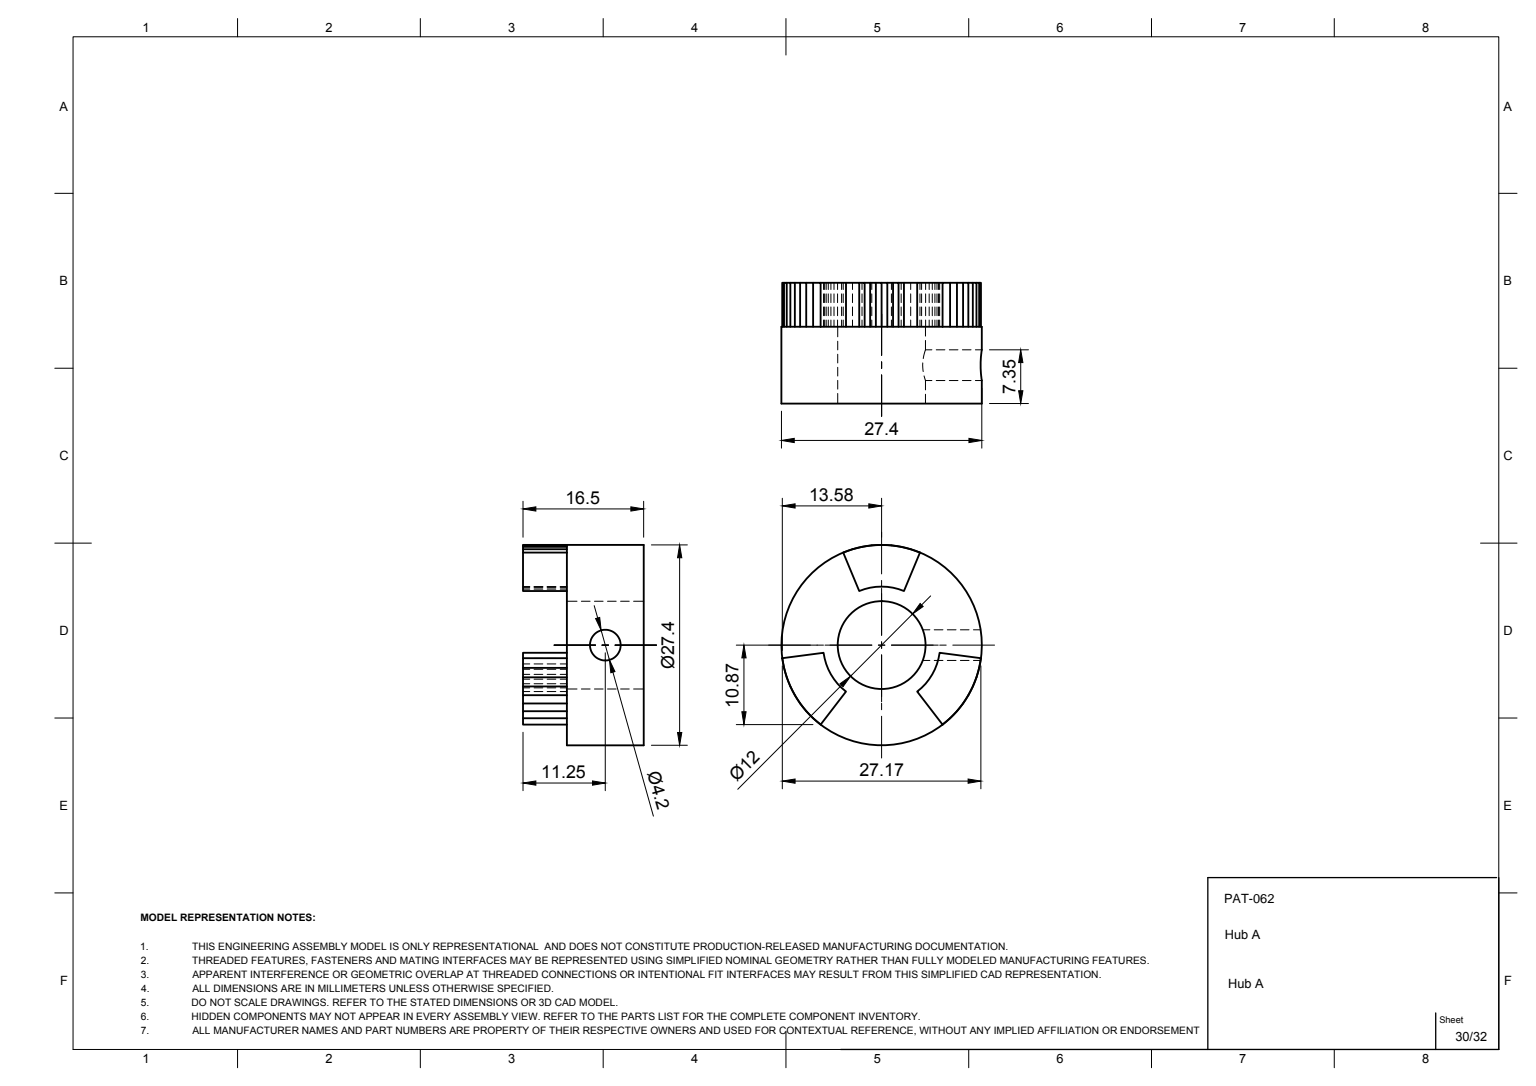
ISO-10303-21;
HEADER;
/* Generated by software containing ST-Developer
 * from STEP Tools, Inc. (www.steptools.com) 
 */

FILE_DESCRIPTION(
/* description */ ('Jaw-coupled motor to shaft test stand'),
/* implementation_level */ '2;1');

FILE_NAME(
/* name */ 'Hub A.step',
/* time_stamp */ '2026-10-27T10:46:06-07:00',
/* author */ (''),
/* organization */ (''),
/* preprocessor_version */ 'ST-DEVELOPER v20.2',
/* originating_system */ 'Autodesk Translation Framework v15.17.0.0',
/* authorisation */ '');

FILE_SCHEMA (('AUTOMOTIVE_DESIGN { 1 0 10303 214 3 1 1 }'));
ENDSEC;

DATA;
#10=MECHANICAL_DESIGN_GEOMETRIC_PRESENTATION_REPRESENTATION('',(#367),#19361);
#267=B_SPLINE_CURVE_WITH_KNOTS('',3,(#17316,#17317,#17318,#17319,#17320,
#17321,#17322,#17323,#17324,#17325,#17326,#17327,#17328,#17329,#17330,#17331,
#17332,#17333),.UNSPECIFIED.,.F.,.F.,(4,2,2,2,2,2,2,2,4),(0.,0.0798638474423531,
0.159727694884706,0.239545993340072,0.319364291795438,0.399182590250804,
0.47900088870617,0.558864736148523,0.638728583590876),.UNSPECIFIED.);
#268=B_SPLINE_CURVE_WITH_KNOTS('',3,(#17334,#17335,#17336,#17337,#17338,
#17339,#17340,#17341,#17342,#17343,#17344,#17345,#17346,#17347,#17348,#17349,
#17350,#17351),.UNSPECIFIED.,.F.,.F.,(4,2,2,2,2,2,2,2,4),(0.638728583590876,
0.718592431033229,0.798456278475582,0.878274576930948,0.958092875386314,
1.03791117384168,1.11772947229705,1.1975933197394,1.27745716718175),
 .UNSPECIFIED.);
#269=B_SPLINE_CURVE_WITH_KNOTS('',3,(#17354,#17355,#17356,#17357,#17358,
#17359,#17360,#17361,#17362,#17363,#17364,#17365,#17366,#17367,#17368,#17369,
#17370,#17371,#17372,#17373,#17374,#17375,#17376,#17377,#17378,#17379,#17380,
#17381,#17382,#17383,#17384,#17385,#17386,#17387),.UNSPECIFIED.,.T.,.F.,
(4,2,2,2,2,2,2,2,2,2,2,2,2,2,2,2,4),(0.,0.079239302416133,0.158478604832266,
0.237716399152057,0.316954193471848,0.39619198779164,0.475429782111431,
0.554669084527564,0.633908386943697,0.71314768935983,0.792386991775963,
0.871624786095754,0.950862580415545,1.03010037473534,1.10933816905513,1.18857747147126,
1.26781677388739),.UNSPECIFIED.);
#302=SHAPE_REPRESENTATION_RELATIONSHIP('SRR','None',#19519,#334);
#334=ADVANCED_BREP_SHAPE_REPRESENTATION('',(#398),#19355);
#367=STYLED_ITEM('',(#19739),#398);
#398=MANIFOLD_SOLID_BREP('Body1',#11013);
#506=FACE_BOUND('',#2012,.T.);
#507=FACE_BOUND('',#2041,.T.);
#508=FACE_BOUND('',#2097,.T.);
#509=FACE_BOUND('',#2099,.T.);
#694=PLANE('',#11869);
#695=PLANE('',#11870);
#696=PLANE('',#11871);
#697=PLANE('',#11872);
#698=PLANE('',#11873);
#699=PLANE('',#11874);
#700=PLANE('',#11875);
#701=PLANE('',#11876);
#702=PLANE('',#11877);
#703=PLANE('',#11878);
#704=PLANE('',#11879);
#705=PLANE('',#11880);
#706=PLANE('',#11881);
#707=PLANE('',#11882);
#708=PLANE('',#11883);
#709=PLANE('',#11884);
#710=PLANE('',#11885);
#711=PLANE('',#11886);
#712=PLANE('',#11887);
#713=PLANE('',#11888);
#714=PLANE('',#11890);
#715=PLANE('',#11892);
#716=PLANE('',#11894);
#717=PLANE('',#11896);
#718=PLANE('',#11898);
#719=PLANE('',#11900);
#720=PLANE('',#11902);
#721=PLANE('',#11904);
#722=PLANE('',#11909);
#723=PLANE('',#11910);
#724=PLANE('',#11911);
#725=PLANE('',#11912);
#726=PLANE('',#11913);
#727=PLANE('',#11914);
#728=PLANE('',#11915);
#729=PLANE('',#11916);
#730=PLANE('',#11917);
#731=PLANE('',#11918);
#732=PLANE('',#11919);
#733=PLANE('',#11920);
#734=PLANE('',#11921);
#735=PLANE('',#11922);
#736=PLANE('',#11923);
#737=PLANE('',#11924);
#738=PLANE('',#11925);
#739=PLANE('',#11926);
#740=PLANE('',#11927);
#741=PLANE('',#11928);
#742=PLANE('',#11930);
#743=PLANE('',#11932);
#744=PLANE('',#11934);
#745=PLANE('',#11936);
#746=PLANE('',#11938);
#747=PLANE('',#11940);
#748=PLANE('',#11942);
#749=PLANE('',#11944);
#750=PLANE('',#11945);
#751=PLANE('',#11946);
#752=PLANE('',#11947);
#753=PLANE('',#11948);
#754=PLANE('',#11949);
#755=PLANE('',#11950);
#756=PLANE('',#11951);
#757=PLANE('',#11952);
#758=PLANE('',#11953);
#759=PLANE('',#11954);
#760=PLANE('',#11955);
#761=PLANE('',#11956);
#762=PLANE('',#11957);
#763=PLANE('',#11958);
#764=PLANE('',#11959);
#765=PLANE('',#11960);
#766=PLANE('',#11961);
#767=PLANE('',#11962);
#768=PLANE('',#11963);
#769=PLANE('',#11965);
#770=PLANE('',#11967);
#771=PLANE('',#11969);
#772=PLANE('',#11971);
#773=PLANE('',#11973);
#774=PLANE('',#11975);
#775=PLANE('',#11977);
#776=PLANE('',#11981);
#1287=FACE_OUTER_BOUND('',#2010,.T.);
#1288=FACE_OUTER_BOUND('',#2011,.T.);
#1289=FACE_OUTER_BOUND('',#2013,.T.);
#1290=FACE_OUTER_BOUND('',#2014,.T.);
#1291=FACE_OUTER_BOUND('',#2015,.T.);
#1292=FACE_OUTER_BOUND('',#2016,.T.);
#1293=FACE_OUTER_BOUND('',#2017,.T.);
#1294=FACE_OUTER_BOUND('',#2018,.T.);
#1295=FACE_OUTER_BOUND('',#2019,.T.);
#1296=FACE_OUTER_BOUND('',#2020,.T.);
#1297=FACE_OUTER_BOUND('',#2021,.T.);
#1298=FACE_OUTER_BOUND('',#2022,.T.);
#1299=FACE_OUTER_BOUND('',#2023,.T.);
#1300=FACE_OUTER_BOUND('',#2024,.T.);
#1301=FACE_OUTER_BOUND('',#2025,.T.);
#1302=FACE_OUTER_BOUND('',#2026,.T.);
#1303=FACE_OUTER_BOUND('',#2027,.T.);
#1304=FACE_OUTER_BOUND('',#2028,.T.);
#1305=FACE_OUTER_BOUND('',#2029,.T.);
#1306=FACE_OUTER_BOUND('',#2030,.T.);
#1307=FACE_OUTER_BOUND('',#2031,.T.);
#1308=FACE_OUTER_BOUND('',#2032,.T.);
#1309=FACE_OUTER_BOUND('',#2033,.T.);
#1310=FACE_OUTER_BOUND('',#2034,.T.);
#1311=FACE_OUTER_BOUND('',#2035,.T.);
#1312=FACE_OUTER_BOUND('',#2036,.T.);
#1313=FACE_OUTER_BOUND('',#2037,.T.);
#1314=FACE_OUTER_BOUND('',#2038,.T.);
#1315=FACE_OUTER_BOUND('',#2039,.T.);
#1316=FACE_OUTER_BOUND('',#2040,.T.);
#1317=FACE_OUTER_BOUND('',#2042,.T.);
#1318=FACE_OUTER_BOUND('',#2043,.T.);
#1319=FACE_OUTER_BOUND('',#2044,.T.);
#1320=FACE_OUTER_BOUND('',#2045,.T.);
#1321=FACE_OUTER_BOUND('',#2046,.T.);
#1322=FACE_OUTER_BOUND('',#2047,.T.);
#1323=FACE_OUTER_BOUND('',#2048,.T.);
#1324=FACE_OUTER_BOUND('',#2049,.T.);
#1325=FACE_OUTER_BOUND('',#2050,.T.);
#1326=FACE_OUTER_BOUND('',#2051,.T.);
#1327=FACE_OUTER_BOUND('',#2052,.T.);
#1328=FACE_OUTER_BOUND('',#2053,.T.);
#1329=FACE_OUTER_BOUND('',#2054,.T.);
#1330=FACE_OUTER_BOUND('',#2055,.T.);
#1331=FACE_OUTER_BOUND('',#2056,.T.);
#1332=FACE_OUTER_BOUND('',#2057,.T.);
#1333=FACE_OUTER_BOUND('',#2058,.T.);
#1334=FACE_OUTER_BOUND('',#2059,.T.);
#1335=FACE_OUTER_BOUND('',#2060,.T.);
#1336=FACE_OUTER_BOUND('',#2061,.T.);
#1337=FACE_OUTER_BOUND('',#2062,.T.);
#1338=FACE_OUTER_BOUND('',#2063,.T.);
#1339=FACE_OUTER_BOUND('',#2064,.T.);
#1340=FACE_OUTER_BOUND('',#2065,.T.);
#1341=FACE_OUTER_BOUND('',#2066,.T.);
#1342=FACE_OUTER_BOUND('',#2067,.T.);
#1343=FACE_OUTER_BOUND('',#2068,.T.);
#1344=FACE_OUTER_BOUND('',#2069,.T.);
#1345=FACE_OUTER_BOUND('',#2070,.T.);
#1346=FACE_OUTER_BOUND('',#2071,.T.);
#1347=FACE_OUTER_BOUND('',#2072,.T.);
#1348=FACE_OUTER_BOUND('',#2073,.T.);
#1349=FACE_OUTER_BOUND('',#2074,.T.);
#1350=FACE_OUTER_BOUND('',#2075,.T.);
#1351=FACE_OUTER_BOUND('',#2076,.T.);
#1352=FACE_OUTER_BOUND('',#2077,.T.);
#1353=FACE_OUTER_BOUND('',#2078,.T.);
#1354=FACE_OUTER_BOUND('',#2079,.T.);
#1355=FACE_OUTER_BOUND('',#2080,.T.);
#1356=FACE_OUTER_BOUND('',#2081,.T.);
#1357=FACE_OUTER_BOUND('',#2082,.T.);
#1358=FACE_OUTER_BOUND('',#2083,.T.);
#1359=FACE_OUTER_BOUND('',#2084,.T.);
#1360=FACE_OUTER_BOUND('',#2085,.T.);
#1361=FACE_OUTER_BOUND('',#2086,.T.);
#1362=FACE_OUTER_BOUND('',#2087,.T.);
#1363=FACE_OUTER_BOUND('',#2088,.T.);
#1364=FACE_OUTER_BOUND('',#2089,.T.);
#1365=FACE_OUTER_BOUND('',#2090,.T.);
#1366=FACE_OUTER_BOUND('',#2091,.T.);
#1367=FACE_OUTER_BOUND('',#2092,.T.);
#1368=FACE_OUTER_BOUND('',#2093,.T.);
#1369=FACE_OUTER_BOUND('',#2094,.T.);
#1370=FACE_OUTER_BOUND('',#2095,.T.);
#1371=FACE_OUTER_BOUND('',#2096,.T.);
#1372=FACE_OUTER_BOUND('',#2098,.T.);
#2010=EDGE_LOOP('',(#8474,#8475,#8476,#8477,#8478));
#2011=EDGE_LOOP('',(#8479,#8480,#8481,#8482));
#2012=EDGE_LOOP('',(#8483,#8484));
#2013=EDGE_LOOP('',(#8485,#8486,#8487,#8488));
#2014=EDGE_LOOP('',(#8489,#8490,#8491,#8492));
#2015=EDGE_LOOP('',(#8493,#8494,#8495,#8496));
#2016=EDGE_LOOP('',(#8497,#8498,#8499,#8500));
#2017=EDGE_LOOP('',(#8501,#8502,#8503,#8504));
#2018=EDGE_LOOP('',(#8505,#8506,#8507,#8508));
#2019=EDGE_LOOP('',(#8509,#8510,#8511,#8512));
#2020=EDGE_LOOP('',(#8513,#8514,#8515,#8516));
#2021=EDGE_LOOP('',(#8517,#8518,#8519,#8520));
#2022=EDGE_LOOP('',(#8521,#8522,#8523,#8524));
#2023=EDGE_LOOP('',(#8525,#8526,#8527,#8528));
#2024=EDGE_LOOP('',(#8529,#8530,#8531,#8532));
#2025=EDGE_LOOP('',(#8533,#8534,#8535,#8536));
#2026=EDGE_LOOP('',(#8537,#8538,#8539,#8540));
#2027=EDGE_LOOP('',(#8541,#8542,#8543,#8544));
#2028=EDGE_LOOP('',(#8545,#8546,#8547,#8548));
#2029=EDGE_LOOP('',(#8549,#8550,#8551,#8552));
#2030=EDGE_LOOP('',(#8553,#8554,#8555,#8556));
#2031=EDGE_LOOP('',(#8557,#8558,#8559,#8560,#8561,#8562,#8563,#8564,#8565,
#8566,#8567,#8568,#8569,#8570,#8571,#8572,#8573,#8574));
#2032=EDGE_LOOP('',(#8575,#8576));
#2033=EDGE_LOOP('',(#8577,#8578));
#2034=EDGE_LOOP('',(#8579,#8580));
#2035=EDGE_LOOP('',(#8581,#8582));
#2036=EDGE_LOOP('',(#8583,#8584));
#2037=EDGE_LOOP('',(#8585,#8586));
#2038=EDGE_LOOP('',(#8587,#8588));
#2039=EDGE_LOOP('',(#8589,#8590));
#2040=EDGE_LOOP('',(#8591,#8592,#8593,#8594,#8595,#8596,#8597,#8598,#8599,
#8600,#8601,#8602,#8603,#8604,#8605,#8606,#8607,#8608,#8609,#8610,#8611,
#8612,#8613,#8614,#8615,#8616,#8617,#8618,#8619,#8620,#8621,#8622,#8623,
#8624));
#2041=EDGE_LOOP('',(#8625));
#2042=EDGE_LOOP('',(#8626,#8627,#8628,#8629));
#2043=EDGE_LOOP('',(#8630,#8631,#8632,#8633));
#2044=EDGE_LOOP('',(#8634,#8635,#8636,#8637));
#2045=EDGE_LOOP('',(#8638,#8639,#8640,#8641));
#2046=EDGE_LOOP('',(#8642,#8643,#8644,#8645));
#2047=EDGE_LOOP('',(#8646,#8647,#8648,#8649));
#2048=EDGE_LOOP('',(#8650,#8651,#8652,#8653));
#2049=EDGE_LOOP('',(#8654,#8655,#8656,#8657));
#2050=EDGE_LOOP('',(#8658,#8659,#8660,#8661));
#2051=EDGE_LOOP('',(#8662,#8663,#8664,#8665));
#2052=EDGE_LOOP('',(#8666,#8667,#8668,#8669));
#2053=EDGE_LOOP('',(#8670,#8671,#8672,#8673));
#2054=EDGE_LOOP('',(#8674,#8675,#8676,#8677));
#2055=EDGE_LOOP('',(#8678,#8679,#8680,#8681));
#2056=EDGE_LOOP('',(#8682,#8683,#8684,#8685));
#2057=EDGE_LOOP('',(#8686,#8687,#8688,#8689));
#2058=EDGE_LOOP('',(#8690,#8691,#8692,#8693));
#2059=EDGE_LOOP('',(#8694,#8695,#8696,#8697));
#2060=EDGE_LOOP('',(#8698,#8699,#8700,#8701,#8702,#8703,#8704,#8705,#8706,
#8707,#8708,#8709,#8710,#8711,#8712,#8713,#8714,#8715));
#2061=EDGE_LOOP('',(#8716,#8717));
#2062=EDGE_LOOP('',(#8718,#8719));
#2063=EDGE_LOOP('',(#8720,#8721));
#2064=EDGE_LOOP('',(#8722,#8723));
#2065=EDGE_LOOP('',(#8724,#8725));
#2066=EDGE_LOOP('',(#8726,#8727));
#2067=EDGE_LOOP('',(#8728,#8729));
#2068=EDGE_LOOP('',(#8730,#8731));
#2069=EDGE_LOOP('',(#8732,#8733,#8734,#8735));
#2070=EDGE_LOOP('',(#8736,#8737,#8738,#8739));
#2071=EDGE_LOOP('',(#8740,#8741,#8742,#8743));
#2072=EDGE_LOOP('',(#8744,#8745,#8746,#8747));
#2073=EDGE_LOOP('',(#8748,#8749,#8750,#8751));
#2074=EDGE_LOOP('',(#8752,#8753,#8754,#8755));
#2075=EDGE_LOOP('',(#8756,#8757,#8758,#8759));
#2076=EDGE_LOOP('',(#8760,#8761,#8762,#8763));
#2077=EDGE_LOOP('',(#8764,#8765,#8766,#8767));
#2078=EDGE_LOOP('',(#8768,#8769,#8770,#8771));
#2079=EDGE_LOOP('',(#8772,#8773,#8774,#8775));
#2080=EDGE_LOOP('',(#8776,#8777,#8778,#8779));
#2081=EDGE_LOOP('',(#8780,#8781,#8782,#8783));
#2082=EDGE_LOOP('',(#8784,#8785,#8786,#8787));
#2083=EDGE_LOOP('',(#8788,#8789,#8790,#8791));
#2084=EDGE_LOOP('',(#8792,#8793,#8794,#8795));
#2085=EDGE_LOOP('',(#8796,#8797,#8798,#8799));
#2086=EDGE_LOOP('',(#8800,#8801,#8802,#8803));
#2087=EDGE_LOOP('',(#8804,#8805,#8806,#8807,#8808,#8809,#8810,#8811,#8812,
#8813,#8814,#8815,#8816,#8817,#8818,#8819,#8820,#8821));
#2088=EDGE_LOOP('',(#8822,#8823));
#2089=EDGE_LOOP('',(#8824,#8825));
#2090=EDGE_LOOP('',(#8826,#8827));
#2091=EDGE_LOOP('',(#8828,#8829));
#2092=EDGE_LOOP('',(#8830,#8831));
#2093=EDGE_LOOP('',(#8832,#8833));
#2094=EDGE_LOOP('',(#8834,#8835));
#2095=EDGE_LOOP('',(#8836,#8837));
#2096=EDGE_LOOP('',(#8838,#8839,#8840,#8841,#8842,#8843,#8844,#8845,#8846,
#8847,#8848,#8849,#8850,#8851,#8852,#8853,#8854,#8855,#8856,#8857,#8858,
#8859,#8860,#8861,#8862,#8863,#8864,#8865,#8866,#8867,#8868));
#2097=EDGE_LOOP('',(#8869));
#2098=EDGE_LOOP('',(#8870));
#2099=EDGE_LOOP('',(#8871));
#2731=LINE('',#17353,#3884);
#2732=LINE('',#17392,#3885);
#2733=LINE('',#17397,#3886);
#2734=LINE('',#17399,#3887);
#2735=LINE('',#17401,#3888);
#2736=LINE('',#17402,#3889);
#2737=LINE('',#17405,#3890);
#2738=LINE('',#17407,#3891);
#2739=LINE('',#17408,#3892);
#2740=LINE('',#17411,#3893);
#2741=LINE('',#17413,#3894);
#2742=LINE('',#17414,#3895);
#2743=LINE('',#17417,#3896);
#2744=LINE('',#17419,#3897);
#2745=LINE('',#17420,#3898);
#2746=LINE('',#17423,#3899);
#2747=LINE('',#17425,#3900);
#2748=LINE('',#17426,#3901);
#2749=LINE('',#17429,#3902);
#2750=LINE('',#17431,#3903);
#2751=LINE('',#17432,#3904);
#2752=LINE('',#17435,#3905);
#2753=LINE('',#17437,#3906);
#2754=LINE('',#17438,#3907);
#2755=LINE('',#17441,#3908);
#2756=LINE('',#17443,#3909);
#2757=LINE('',#17444,#3910);
#2758=LINE('',#17447,#3911);
#2759=LINE('',#17449,#3912);
#2760=LINE('',#17450,#3913);
#2761=LINE('',#17453,#3914);
#2762=LINE('',#17455,#3915);
#2763=LINE('',#17456,#3916);
#2764=LINE('',#17459,#3917);
#2765=LINE('',#17461,#3918);
#2766=LINE('',#17462,#3919);
#2767=LINE('',#17465,#3920);
#2768=LINE('',#17467,#3921);
#2769=LINE('',#17468,#3922);
#2770=LINE('',#17471,#3923);
#2771=LINE('',#17473,#3924);
#2772=LINE('',#17474,#3925);
#2773=LINE('',#17477,#3926);
#2774=LINE('',#17479,#3927);
#2775=LINE('',#17480,#3928);
#2776=LINE('',#17483,#3929);
#2777=LINE('',#17485,#3930);
#2778=LINE('',#17486,#3931);
#2779=LINE('',#17489,#3932);
#2780=LINE('',#17491,#3933);
#2781=LINE('',#17492,#3934);
#2782=LINE('',#17495,#3935);
#2783=LINE('',#17497,#3936);
#2784=LINE('',#17498,#3937);
#2785=LINE('',#17500,#3938);
#2786=LINE('',#17501,#3939);
#2787=LINE('',#17523,#3940);
#2788=LINE('',#17525,#3941);
#2789=LINE('',#17527,#3942);
#2790=LINE('',#17529,#3943);
#2791=LINE('',#17531,#3944);
#2792=LINE('',#17533,#3945);
#2793=LINE('',#17535,#3946);
#2794=LINE('',#17537,#3947);
#2795=LINE('',#17539,#3948);
#2796=LINE('',#17541,#3949);
#2797=LINE('',#17545,#3950);
#2798=LINE('',#17547,#3951);
#2799=LINE('',#17549,#3952);
#2800=LINE('',#17551,#3953);
#2801=LINE('',#17553,#3954);
#2802=LINE('',#17555,#3955);
#2803=LINE('',#17557,#3956);
#2804=LINE('',#17559,#3957);
#2805=LINE('',#17561,#3958);
#2806=LINE('',#17563,#3959);
#2807=LINE('',#17570,#3960);
#2808=LINE('',#17571,#3961);
#2809=LINE('',#17573,#3962);
#2810=LINE('',#17574,#3963);
#2811=LINE('',#17577,#3964);
#2812=LINE('',#17579,#3965);
#2813=LINE('',#17580,#3966);
#2814=LINE('',#17583,#3967);
#2815=LINE('',#17585,#3968);
#2816=LINE('',#17586,#3969);
#2817=LINE('',#17589,#3970);
#2818=LINE('',#17591,#3971);
#2819=LINE('',#17592,#3972);
#2820=LINE('',#17595,#3973);
#2821=LINE('',#17597,#3974);
#2822=LINE('',#17598,#3975);
#2823=LINE('',#17601,#3976);
#2824=LINE('',#17603,#3977);
#2825=LINE('',#17604,#3978);
#2826=LINE('',#17607,#3979);
#2827=LINE('',#17609,#3980);
#2828=LINE('',#17610,#3981);
#2829=LINE('',#17613,#3982);
#2830=LINE('',#17614,#3983);
#2831=LINE('',#17615,#3984);
#2832=LINE('',#17618,#3985);
#2833=LINE('',#17619,#3986);
#2834=LINE('',#17622,#3987);
#2835=LINE('',#17623,#3988);
#2836=LINE('',#17626,#3989);
#2837=LINE('',#17627,#3990);
#2838=LINE('',#17630,#3991);
#2839=LINE('',#17631,#3992);
#2840=LINE('',#17634,#3993);
#2841=LINE('',#17635,#3994);
#2842=LINE('',#17638,#3995);
#2843=LINE('',#17639,#3996);
#2844=LINE('',#17642,#3997);
#2845=LINE('',#17643,#3998);
#2846=LINE('',#17646,#3999);
#2847=LINE('',#17647,#4000);
#2848=LINE('',#17650,#4001);
#2849=LINE('',#17651,#4002);
#2850=LINE('',#17653,#4003);
#2851=LINE('',#17674,#4004);
#2852=LINE('',#17675,#4005);
#2853=LINE('',#17677,#4006);
#2854=LINE('',#17678,#4007);
#2855=LINE('',#17681,#4008);
#2856=LINE('',#17683,#4009);
#2857=LINE('',#17684,#4010);
#2858=LINE('',#17687,#4011);
#2859=LINE('',#17689,#4012);
#2860=LINE('',#17690,#4013);
#2861=LINE('',#17693,#4014);
#2862=LINE('',#17695,#4015);
#2863=LINE('',#17696,#4016);
#2864=LINE('',#17699,#4017);
#2865=LINE('',#17701,#4018);
#2866=LINE('',#17702,#4019);
#2867=LINE('',#17705,#4020);
#2868=LINE('',#17707,#4021);
#2869=LINE('',#17708,#4022);
#2870=LINE('',#17711,#4023);
#2871=LINE('',#17713,#4024);
#2872=LINE('',#17714,#4025);
#2873=LINE('',#17717,#4026);
#2874=LINE('',#17718,#4027);
#2875=LINE('',#17719,#4028);
#2876=LINE('',#17722,#4029);
#2877=LINE('',#17723,#4030);
#2878=LINE('',#17726,#4031);
#2879=LINE('',#17727,#4032);
#2880=LINE('',#17730,#4033);
#2881=LINE('',#17731,#4034);
#2882=LINE('',#17734,#4035);
#2883=LINE('',#17735,#4036);
#2884=LINE('',#17738,#4037);
#2885=LINE('',#17739,#4038);
#2886=LINE('',#17742,#4039);
#2887=LINE('',#17743,#4040);
#2888=LINE('',#17746,#4041);
#2889=LINE('',#17747,#4042);
#2890=LINE('',#17750,#4043);
#2891=LINE('',#17751,#4044);
#2892=LINE('',#17754,#4045);
#2893=LINE('',#17755,#4046);
#2894=LINE('',#17757,#4047);
#2895=LINE('',#17778,#4048);
#3884=VECTOR('',#13682,0.21);
#3885=VECTOR('',#13687,0.6);
#3886=VECTOR('',#13692,1.);
#3887=VECTOR('',#13693,1.);
#3888=VECTOR('',#13694,1.);
#3889=VECTOR('',#13695,1.);
#3890=VECTOR('',#13698,1.);
#3891=VECTOR('',#13699,1.);
#3892=VECTOR('',#13700,1.);
#3893=VECTOR('',#13703,1.);
#3894=VECTOR('',#13704,1.);
#3895=VECTOR('',#13705,1.);
#3896=VECTOR('',#13708,1.);
#3897=VECTOR('',#13709,1.);
#3898=VECTOR('',#13710,1.);
#3899=VECTOR('',#13713,1.);
#3900=VECTOR('',#13714,1.);
#3901=VECTOR('',#13715,1.);
#3902=VECTOR('',#13718,1.);
#3903=VECTOR('',#13719,1.);
#3904=VECTOR('',#13720,1.);
#3905=VECTOR('',#13723,1.);
#3906=VECTOR('',#13724,1.);
#3907=VECTOR('',#13725,1.);
#3908=VECTOR('',#13728,1.);
#3909=VECTOR('',#13729,1.);
#3910=VECTOR('',#13730,1.);
#3911=VECTOR('',#13733,1.);
#3912=VECTOR('',#13734,1.);
#3913=VECTOR('',#13735,1.);
#3914=VECTOR('',#13738,1.);
#3915=VECTOR('',#13739,1.);
#3916=VECTOR('',#13740,1.);
#3917=VECTOR('',#13743,1.);
#3918=VECTOR('',#13744,1.);
#3919=VECTOR('',#13745,1.);
#3920=VECTOR('',#13748,1.);
#3921=VECTOR('',#13749,1.);
#3922=VECTOR('',#13750,1.);
#3923=VECTOR('',#13753,1.);
#3924=VECTOR('',#13754,1.);
#3925=VECTOR('',#13755,1.);
#3926=VECTOR('',#13758,1.);
#3927=VECTOR('',#13759,1.);
#3928=VECTOR('',#13760,1.);
#3929=VECTOR('',#13763,1.);
#3930=VECTOR('',#13764,1.);
#3931=VECTOR('',#13765,1.);
#3932=VECTOR('',#13768,1.);
#3933=VECTOR('',#13769,1.);
#3934=VECTOR('',#13770,1.);
#3935=VECTOR('',#13773,1.);
#3936=VECTOR('',#13774,1.);
#3937=VECTOR('',#13775,1.);
#3938=VECTOR('',#13778,1.);
#3939=VECTOR('',#13779,1.);
#3940=VECTOR('',#13818,1.);
#3941=VECTOR('',#13819,1.);
#3942=VECTOR('',#13820,1.);
#3943=VECTOR('',#13821,1.);
#3944=VECTOR('',#13822,1.);
#3945=VECTOR('',#13823,1.);
#3946=VECTOR('',#13824,1.);
#3947=VECTOR('',#13825,1.);
#3948=VECTOR('',#13826,1.);
#3949=VECTOR('',#13827,1.);
#3950=VECTOR('',#13830,1.);
#3951=VECTOR('',#13831,1.);
#3952=VECTOR('',#13832,1.);
#3953=VECTOR('',#13833,1.);
#3954=VECTOR('',#13834,1.);
#3955=VECTOR('',#13835,1.);
#3956=VECTOR('',#13836,1.);
#3957=VECTOR('',#13837,1.);
#3958=VECTOR('',#13838,1.);
#3959=VECTOR('',#13839,1.);
#3960=VECTOR('',#13846,1.);
#3961=VECTOR('',#13847,1.);
#3962=VECTOR('',#13848,1.);
#3963=VECTOR('',#13849,1.);
#3964=VECTOR('',#13852,1.);
#3965=VECTOR('',#13853,1.);
#3966=VECTOR('',#13854,1.);
#3967=VECTOR('',#13857,1.);
#3968=VECTOR('',#13858,1.);
#3969=VECTOR('',#13859,1.);
#3970=VECTOR('',#13862,1.);
#3971=VECTOR('',#13863,1.);
#3972=VECTOR('',#13864,1.);
#3973=VECTOR('',#13867,1.);
#3974=VECTOR('',#13868,1.);
#3975=VECTOR('',#13869,1.);
#3976=VECTOR('',#13872,1.);
#3977=VECTOR('',#13873,1.);
#3978=VECTOR('',#13874,1.);
#3979=VECTOR('',#13877,1.);
#3980=VECTOR('',#13878,1.);
#3981=VECTOR('',#13879,1.);
#3982=VECTOR('',#13882,1.);
#3983=VECTOR('',#13883,1.);
#3984=VECTOR('',#13884,1.);
#3985=VECTOR('',#13887,1.);
#3986=VECTOR('',#13888,1.);
#3987=VECTOR('',#13891,1.);
#3988=VECTOR('',#13892,1.);
#3989=VECTOR('',#13895,1.);
#3990=VECTOR('',#13896,1.);
#3991=VECTOR('',#13899,1.);
#3992=VECTOR('',#13900,1.);
#3993=VECTOR('',#13903,1.);
#3994=VECTOR('',#13904,1.);
#3995=VECTOR('',#13907,1.);
#3996=VECTOR('',#13908,1.);
#3997=VECTOR('',#13911,1.);
#3998=VECTOR('',#13912,1.);
#3999=VECTOR('',#13915,1.);
#4000=VECTOR('',#13916,1.);
#4001=VECTOR('',#13919,1.);
#4002=VECTOR('',#13920,1.);
#4003=VECTOR('',#13923,1.);
#4004=VECTOR('',#13960,1.);
#4005=VECTOR('',#13961,1.);
#4006=VECTOR('',#13962,1.);
#4007=VECTOR('',#13963,1.);
#4008=VECTOR('',#13966,1.);
#4009=VECTOR('',#13967,1.);
#4010=VECTOR('',#13968,1.);
#4011=VECTOR('',#13971,1.);
#4012=VECTOR('',#13972,1.);
#4013=VECTOR('',#13973,1.);
#4014=VECTOR('',#13976,1.);
#4015=VECTOR('',#13977,1.);
#4016=VECTOR('',#13978,1.);
#4017=VECTOR('',#13981,1.);
#4018=VECTOR('',#13982,1.);
#4019=VECTOR('',#13983,1.);
#4020=VECTOR('',#13986,1.);
#4021=VECTOR('',#13987,1.);
#4022=VECTOR('',#13988,1.);
#4023=VECTOR('',#13991,1.);
#4024=VECTOR('',#13992,1.);
#4025=VECTOR('',#13993,1.);
#4026=VECTOR('',#13996,1.);
#4027=VECTOR('',#13997,1.);
#4028=VECTOR('',#13998,1.);
#4029=VECTOR('',#14001,1.);
#4030=VECTOR('',#14002,1.);
#4031=VECTOR('',#14005,1.);
#4032=VECTOR('',#14006,1.);
#4033=VECTOR('',#14009,1.);
#4034=VECTOR('',#14010,1.);
#4035=VECTOR('',#14013,1.);
#4036=VECTOR('',#14014,1.);
#4037=VECTOR('',#14017,1.);
#4038=VECTOR('',#14018,1.);
#4039=VECTOR('',#14021,1.);
#4040=VECTOR('',#14022,1.);
#4041=VECTOR('',#14025,1.);
#4042=VECTOR('',#14026,1.);
#4043=VECTOR('',#14029,1.);
#4044=VECTOR('',#14030,1.);
#4045=VECTOR('',#14033,1.);
#4046=VECTOR('',#14034,1.);
#4047=VECTOR('',#14037,1.);
#4048=VECTOR('',#14076,1.37);
#4849=CIRCLE('',#11867,0.6);
#4850=CIRCLE('',#11868,0.6);
#4851=CIRCLE('',#11889,1.37);
#4852=CIRCLE('',#11891,1.37);
#4853=CIRCLE('',#11893,1.37);
#4854=CIRCLE('',#11895,1.37);
#4855=CIRCLE('',#11897,1.37);
#4856=CIRCLE('',#11899,1.37);
#4857=CIRCLE('',#11901,1.37);
#4858=CIRCLE('',#11903,1.37);
#4859=CIRCLE('',#11905,1.37);
#4860=CIRCLE('',#11906,1.37);
#4861=CIRCLE('',#11907,1.37);
#4862=CIRCLE('',#11908,1.37);
#4863=CIRCLE('',#11929,1.37);
#4864=CIRCLE('',#11931,1.37);
#4865=CIRCLE('',#11933,1.37);
#4866=CIRCLE('',#11935,1.37);
#4867=CIRCLE('',#11937,1.37);
#4868=CIRCLE('',#11939,1.37);
#4869=CIRCLE('',#11941,1.37);
#4870=CIRCLE('',#11943,1.37);
#4871=CIRCLE('',#11964,1.37);
#4872=CIRCLE('',#11966,1.37);
#4873=CIRCLE('',#11968,1.37);
#4874=CIRCLE('',#11970,1.37);
#4875=CIRCLE('',#11972,1.37);
#4876=CIRCLE('',#11974,1.37);
#4877=CIRCLE('',#11976,1.37);
#4878=CIRCLE('',#11978,1.37);
#4879=CIRCLE('',#11980,1.37);
#5325=VERTEX_POINT('',#17314);
#5326=VERTEX_POINT('',#17315);
#5327=VERTEX_POINT('',#17352);
#5328=VERTEX_POINT('',#17389);
#5329=VERTEX_POINT('',#17391);
#5330=VERTEX_POINT('',#17395);
#5331=VERTEX_POINT('',#17396);
#5332=VERTEX_POINT('',#17398);
#5333=VERTEX_POINT('',#17400);
#5334=VERTEX_POINT('',#17404);
#5335=VERTEX_POINT('',#17406);
#5336=VERTEX_POINT('',#17410);
#5337=VERTEX_POINT('',#17412);
#5338=VERTEX_POINT('',#17416);
#5339=VERTEX_POINT('',#17418);
#5340=VERTEX_POINT('',#17422);
#5341=VERTEX_POINT('',#17424);
#5342=VERTEX_POINT('',#17428);
#5343=VERTEX_POINT('',#17430);
#5344=VERTEX_POINT('',#17434);
#5345=VERTEX_POINT('',#17436);
#5346=VERTEX_POINT('',#17440);
#5347=VERTEX_POINT('',#17442);
#5348=VERTEX_POINT('',#17446);
#5349=VERTEX_POINT('',#17448);
#5350=VERTEX_POINT('',#17452);
#5351=VERTEX_POINT('',#17454);
#5352=VERTEX_POINT('',#17458);
#5353=VERTEX_POINT('',#17460);
#5354=VERTEX_POINT('',#17464);
#5355=VERTEX_POINT('',#17466);
#5356=VERTEX_POINT('',#17470);
#5357=VERTEX_POINT('',#17472);
#5358=VERTEX_POINT('',#17476);
#5359=VERTEX_POINT('',#17478);
#5360=VERTEX_POINT('',#17482);
#5361=VERTEX_POINT('',#17484);
#5362=VERTEX_POINT('',#17488);
#5363=VERTEX_POINT('',#17490);
#5364=VERTEX_POINT('',#17494);
#5365=VERTEX_POINT('',#17496);
#5366=VERTEX_POINT('',#17520);
#5367=VERTEX_POINT('',#17522);
#5368=VERTEX_POINT('',#17524);
#5369=VERTEX_POINT('',#17526);
#5370=VERTEX_POINT('',#17528);
#5371=VERTEX_POINT('',#17530);
#5372=VERTEX_POINT('',#17532);
#5373=VERTEX_POINT('',#17534);
#5374=VERTEX_POINT('',#17536);
#5375=VERTEX_POINT('',#17538);
#5376=VERTEX_POINT('',#17540);
#5377=VERTEX_POINT('',#17542);
#5378=VERTEX_POINT('',#17544);
#5379=VERTEX_POINT('',#17546);
#5380=VERTEX_POINT('',#17548);
#5381=VERTEX_POINT('',#17550);
#5382=VERTEX_POINT('',#17552);
#5383=VERTEX_POINT('',#17554);
#5384=VERTEX_POINT('',#17556);
#5385=VERTEX_POINT('',#17558);
#5386=VERTEX_POINT('',#17560);
#5387=VERTEX_POINT('',#17562);
#5388=VERTEX_POINT('',#17564);
#5389=VERTEX_POINT('',#17568);
#5390=VERTEX_POINT('',#17569);
#5391=VERTEX_POINT('',#17572);
#5392=VERTEX_POINT('',#17576);
#5393=VERTEX_POINT('',#17578);
#5394=VERTEX_POINT('',#17582);
#5395=VERTEX_POINT('',#17584);
#5396=VERTEX_POINT('',#17588);
#5397=VERTEX_POINT('',#17590);
#5398=VERTEX_POINT('',#17594);
#5399=VERTEX_POINT('',#17596);
#5400=VERTEX_POINT('',#17600);
#5401=VERTEX_POINT('',#17602);
#5402=VERTEX_POINT('',#17606);
#5403=VERTEX_POINT('',#17608);
#5404=VERTEX_POINT('',#17612);
#5405=VERTEX_POINT('',#17617);
#5406=VERTEX_POINT('',#17621);
#5407=VERTEX_POINT('',#17625);
#5408=VERTEX_POINT('',#17629);
#5409=VERTEX_POINT('',#17633);
#5410=VERTEX_POINT('',#17637);
#5411=VERTEX_POINT('',#17641);
#5412=VERTEX_POINT('',#17645);
#5413=VERTEX_POINT('',#17649);
#5414=VERTEX_POINT('',#17672);
#5415=VERTEX_POINT('',#17673);
#5416=VERTEX_POINT('',#17676);
#5417=VERTEX_POINT('',#17680);
#5418=VERTEX_POINT('',#17682);
#5419=VERTEX_POINT('',#17686);
#5420=VERTEX_POINT('',#17688);
#5421=VERTEX_POINT('',#17692);
#5422=VERTEX_POINT('',#17694);
#5423=VERTEX_POINT('',#17698);
#5424=VERTEX_POINT('',#17700);
#5425=VERTEX_POINT('',#17704);
#5426=VERTEX_POINT('',#17706);
#5427=VERTEX_POINT('',#17710);
#5428=VERTEX_POINT('',#17712);
#5429=VERTEX_POINT('',#17716);
#5430=VERTEX_POINT('',#17721);
#5431=VERTEX_POINT('',#17725);
#5432=VERTEX_POINT('',#17729);
#5433=VERTEX_POINT('',#17733);
#5434=VERTEX_POINT('',#17737);
#5435=VERTEX_POINT('',#17741);
#5436=VERTEX_POINT('',#17745);
#5437=VERTEX_POINT('',#17749);
#5438=VERTEX_POINT('',#17753);
#5439=VERTEX_POINT('',#17776);
#6448=EDGE_CURVE('',#5325,#5326,#267,.T.);
#6449=EDGE_CURVE('',#5326,#5325,#268,.T.);
#6450=EDGE_CURVE('',#5326,#5327,#2731,.T.);
#6451=EDGE_CURVE('',#5327,#5327,#269,.T.);
#6452=EDGE_CURVE('',#5328,#5328,#4849,.T.);
#6453=EDGE_CURVE('',#5328,#5329,#2732,.T.);
#6454=EDGE_CURVE('',#5329,#5329,#4850,.T.);
#6455=EDGE_CURVE('',#5330,#5331,#2733,.T.);
#6456=EDGE_CURVE('',#5330,#5332,#2734,.T.);
#6457=EDGE_CURVE('',#5333,#5332,#2735,.T.);
#6458=EDGE_CURVE('',#5331,#5333,#2736,.T.);
#6459=EDGE_CURVE('',#5331,#5334,#2737,.T.);
#6460=EDGE_CURVE('',#5335,#5333,#2738,.T.);
#6461=EDGE_CURVE('',#5334,#5335,#2739,.T.);
#6462=EDGE_CURVE('',#5334,#5336,#2740,.T.);
#6463=EDGE_CURVE('',#5337,#5335,#2741,.T.);
#6464=EDGE_CURVE('',#5336,#5337,#2742,.T.);
#6465=EDGE_CURVE('',#5336,#5338,#2743,.T.);
#6466=EDGE_CURVE('',#5339,#5337,#2744,.T.);
#6467=EDGE_CURVE('',#5338,#5339,#2745,.T.);
#6468=EDGE_CURVE('',#5338,#5340,#2746,.T.);
#6469=EDGE_CURVE('',#5341,#5339,#2747,.T.);
#6470=EDGE_CURVE('',#5340,#5341,#2748,.T.);
#6471=EDGE_CURVE('',#5340,#5342,#2749,.T.);
#6472=EDGE_CURVE('',#5343,#5341,#2750,.T.);
#6473=EDGE_CURVE('',#5342,#5343,#2751,.T.);
#6474=EDGE_CURVE('',#5342,#5344,#2752,.T.);
#6475=EDGE_CURVE('',#5345,#5343,#2753,.T.);
#6476=EDGE_CURVE('',#5344,#5345,#2754,.T.);
#6477=EDGE_CURVE('',#5344,#5346,#2755,.T.);
#6478=EDGE_CURVE('',#5347,#5345,#2756,.T.);
#6479=EDGE_CURVE('',#5346,#5347,#2757,.T.);
#6480=EDGE_CURVE('',#5346,#5348,#2758,.T.);
#6481=EDGE_CURVE('',#5349,#5347,#2759,.T.);
#6482=EDGE_CURVE('',#5348,#5349,#2760,.T.);
#6483=EDGE_CURVE('',#5348,#5350,#2761,.T.);
#6484=EDGE_CURVE('',#5351,#5349,#2762,.T.);
#6485=EDGE_CURVE('',#5350,#5351,#2763,.T.);
#6486=EDGE_CURVE('',#5350,#5352,#2764,.T.);
#6487=EDGE_CURVE('',#5353,#5351,#2765,.T.);
#6488=EDGE_CURVE('',#5352,#5353,#2766,.T.);
#6489=EDGE_CURVE('',#5352,#5354,#2767,.T.);
#6490=EDGE_CURVE('',#5355,#5353,#2768,.T.);
#6491=EDGE_CURVE('',#5354,#5355,#2769,.T.);
#6492=EDGE_CURVE('',#5354,#5356,#2770,.T.);
#6493=EDGE_CURVE('',#5357,#5355,#2771,.T.);
#6494=EDGE_CURVE('',#5356,#5357,#2772,.T.);
#6495=EDGE_CURVE('',#5356,#5358,#2773,.T.);
#6496=EDGE_CURVE('',#5359,#5357,#2774,.T.);
#6497=EDGE_CURVE('',#5358,#5359,#2775,.T.);
#6498=EDGE_CURVE('',#5358,#5360,#2776,.T.);
#6499=EDGE_CURVE('',#5361,#5359,#2777,.T.);
#6500=EDGE_CURVE('',#5360,#5361,#2778,.T.);
#6501=EDGE_CURVE('',#5360,#5362,#2779,.T.);
#6502=EDGE_CURVE('',#5363,#5361,#2780,.T.);
#6503=EDGE_CURVE('',#5362,#5363,#2781,.T.);
#6504=EDGE_CURVE('',#5362,#5364,#2782,.T.);
#6505=EDGE_CURVE('',#5365,#5363,#2783,.T.);
#6506=EDGE_CURVE('',#5364,#5365,#2784,.T.);
#6507=EDGE_CURVE('',#5364,#5330,#2785,.T.);
#6508=EDGE_CURVE('',#5332,#5365,#2786,.T.);
#6509=EDGE_CURVE('',#5332,#5333,#4851,.T.);
#6510=EDGE_CURVE('',#5333,#5335,#4852,.T.);
#6511=EDGE_CURVE('',#5335,#5337,#4853,.T.);
#6512=EDGE_CURVE('',#5337,#5339,#4854,.T.);
#6513=EDGE_CURVE('',#5339,#5341,#4855,.T.);
#6514=EDGE_CURVE('',#5341,#5343,#4856,.T.);
#6515=EDGE_CURVE('',#5343,#5345,#4857,.T.);
#6516=EDGE_CURVE('',#5345,#5347,#4858,.T.);
#6517=EDGE_CURVE('',#5347,#5366,#4859,.T.);
#6518=EDGE_CURVE('',#5366,#5367,#2787,.T.);
#6519=EDGE_CURVE('',#5367,#5368,#2788,.T.);
#6520=EDGE_CURVE('',#5368,#5369,#2789,.T.);
#6521=EDGE_CURVE('',#5369,#5370,#2790,.T.);
#6522=EDGE_CURVE('',#5370,#5371,#2791,.T.);
#6523=EDGE_CURVE('',#5371,#5372,#2792,.T.);
#6524=EDGE_CURVE('',#5372,#5373,#2793,.T.);
#6525=EDGE_CURVE('',#5373,#5374,#2794,.T.);
#6526=EDGE_CURVE('',#5374,#5375,#2795,.T.);
#6527=EDGE_CURVE('',#5375,#5376,#2796,.T.);
#6528=EDGE_CURVE('',#5376,#5377,#4860,.T.);
#6529=EDGE_CURVE('',#5377,#5378,#2797,.T.);
#6530=EDGE_CURVE('',#5378,#5379,#2798,.T.);
#6531=EDGE_CURVE('',#5379,#5380,#2799,.T.);
#6532=EDGE_CURVE('',#5380,#5381,#2800,.T.);
#6533=EDGE_CURVE('',#5381,#5382,#2801,.T.);
#6534=EDGE_CURVE('',#5382,#5383,#2802,.T.);
#6535=EDGE_CURVE('',#5383,#5384,#2803,.T.);
#6536=EDGE_CURVE('',#5384,#5385,#2804,.T.);
#6537=EDGE_CURVE('',#5385,#5386,#2805,.T.);
#6538=EDGE_CURVE('',#5386,#5387,#2806,.T.);
#6539=EDGE_CURVE('',#5387,#5388,#4861,.T.);
#6540=EDGE_CURVE('',#5388,#5332,#4862,.T.);
#6541=EDGE_CURVE('',#5389,#5390,#2807,.T.);
#6542=EDGE_CURVE('',#5389,#5377,#2808,.T.);
#6543=EDGE_CURVE('',#5391,#5377,#2809,.T.);
#6544=EDGE_CURVE('',#5390,#5391,#2810,.T.);
#6545=EDGE_CURVE('',#5390,#5392,#2811,.T.);
#6546=EDGE_CURVE('',#5393,#5391,#2812,.T.);
#6547=EDGE_CURVE('',#5392,#5393,#2813,.T.);
#6548=EDGE_CURVE('',#5392,#5394,#2814,.T.);
#6549=EDGE_CURVE('',#5395,#5393,#2815,.T.);
#6550=EDGE_CURVE('',#5394,#5395,#2816,.T.);
#6551=EDGE_CURVE('',#5394,#5396,#2817,.T.);
#6552=EDGE_CURVE('',#5397,#5395,#2818,.T.);
#6553=EDGE_CURVE('',#5396,#5397,#2819,.T.);
#6554=EDGE_CURVE('',#5396,#5398,#2820,.T.);
#6555=EDGE_CURVE('',#5399,#5397,#2821,.T.);
#6556=EDGE_CURVE('',#5398,#5399,#2822,.T.);
#6557=EDGE_CURVE('',#5398,#5400,#2823,.T.);
#6558=EDGE_CURVE('',#5401,#5399,#2824,.T.);
#6559=EDGE_CURVE('',#5400,#5401,#2825,.T.);
#6560=EDGE_CURVE('',#5400,#5402,#2826,.T.);
#6561=EDGE_CURVE('',#5403,#5401,#2827,.T.);
#6562=EDGE_CURVE('',#5402,#5403,#2828,.T.);
#6563=EDGE_CURVE('',#5402,#5404,#2829,.T.);
#6564=EDGE_CURVE('',#5387,#5403,#2830,.T.);
#6565=EDGE_CURVE('',#5404,#5387,#2831,.T.);
#6566=EDGE_CURVE('',#5404,#5405,#2832,.T.);
#6567=EDGE_CURVE('',#5405,#5386,#2833,.T.);
#6568=EDGE_CURVE('',#5405,#5406,#2834,.T.);
#6569=EDGE_CURVE('',#5406,#5385,#2835,.T.);
#6570=EDGE_CURVE('',#5406,#5407,#2836,.T.);
#6571=EDGE_CURVE('',#5407,#5384,#2837,.T.);
#6572=EDGE_CURVE('',#5407,#5408,#2838,.T.);
#6573=EDGE_CURVE('',#5408,#5383,#2839,.T.);
#6574=EDGE_CURVE('',#5408,#5409,#2840,.T.);
#6575=EDGE_CURVE('',#5409,#5382,#2841,.T.);
#6576=EDGE_CURVE('',#5409,#5410,#2842,.T.);
#6577=EDGE_CURVE('',#5410,#5381,#2843,.T.);
#6578=EDGE_CURVE('',#5410,#5411,#2844,.T.);
#6579=EDGE_CURVE('',#5411,#5380,#2845,.T.);
#6580=EDGE_CURVE('',#5411,#5412,#2846,.T.);
#6581=EDGE_CURVE('',#5412,#5379,#2847,.T.);
#6582=EDGE_CURVE('',#5412,#5413,#2848,.T.);
#6583=EDGE_CURVE('',#5413,#5378,#2849,.T.);
#6584=EDGE_CURVE('',#5413,#5389,#2850,.T.);
#6585=EDGE_CURVE('',#5377,#5391,#4863,.T.);
#6586=EDGE_CURVE('',#5391,#5393,#4864,.T.);
#6587=EDGE_CURVE('',#5393,#5395,#4865,.T.);
#6588=EDGE_CURVE('',#5395,#5397,#4866,.T.);
#6589=EDGE_CURVE('',#5397,#5399,#4867,.T.);
#6590=EDGE_CURVE('',#5399,#5401,#4868,.T.);
#6591=EDGE_CURVE('',#5401,#5403,#4869,.T.);
#6592=EDGE_CURVE('',#5403,#5387,#4870,.T.);
#6593=EDGE_CURVE('',#5414,#5415,#2851,.T.);
#6594=EDGE_CURVE('',#5414,#5366,#2852,.T.);
#6595=EDGE_CURVE('',#5416,#5366,#2853,.T.);
#6596=EDGE_CURVE('',#5415,#5416,#2854,.T.);
#6597=EDGE_CURVE('',#5415,#5417,#2855,.T.);
#6598=EDGE_CURVE('',#5418,#5416,#2856,.T.);
#6599=EDGE_CURVE('',#5417,#5418,#2857,.T.);
#6600=EDGE_CURVE('',#5417,#5419,#2858,.T.);
#6601=EDGE_CURVE('',#5420,#5418,#2859,.T.);
#6602=EDGE_CURVE('',#5419,#5420,#2860,.T.);
#6603=EDGE_CURVE('',#5419,#5421,#2861,.T.);
#6604=EDGE_CURVE('',#5422,#5420,#2862,.T.);
#6605=EDGE_CURVE('',#5421,#5422,#2863,.T.);
#6606=EDGE_CURVE('',#5421,#5423,#2864,.T.);
#6607=EDGE_CURVE('',#5424,#5422,#2865,.T.);
#6608=EDGE_CURVE('',#5423,#5424,#2866,.T.);
#6609=EDGE_CURVE('',#5423,#5425,#2867,.T.);
#6610=EDGE_CURVE('',#5426,#5424,#2868,.T.);
#6611=EDGE_CURVE('',#5425,#5426,#2869,.T.);
#6612=EDGE_CURVE('',#5425,#5427,#2870,.T.);
#6613=EDGE_CURVE('',#5428,#5426,#2871,.T.);
#6614=EDGE_CURVE('',#5427,#5428,#2872,.T.);
#6615=EDGE_CURVE('',#5427,#5429,#2873,.T.);
#6616=EDGE_CURVE('',#5376,#5428,#2874,.T.);
#6617=EDGE_CURVE('',#5429,#5376,#2875,.T.);
#6618=EDGE_CURVE('',#5429,#5430,#2876,.T.);
#6619=EDGE_CURVE('',#5430,#5375,#2877,.T.);
#6620=EDGE_CURVE('',#5430,#5431,#2878,.T.);
#6621=EDGE_CURVE('',#5431,#5374,#2879,.T.);
#6622=EDGE_CURVE('',#5431,#5432,#2880,.T.);
#6623=EDGE_CURVE('',#5432,#5373,#2881,.T.);
#6624=EDGE_CURVE('',#5432,#5433,#2882,.T.);
#6625=EDGE_CURVE('',#5433,#5372,#2883,.T.);
#6626=EDGE_CURVE('',#5433,#5434,#2884,.T.);
#6627=EDGE_CURVE('',#5434,#5371,#2885,.T.);
#6628=EDGE_CURVE('',#5434,#5435,#2886,.T.);
#6629=EDGE_CURVE('',#5435,#5370,#2887,.T.);
#6630=EDGE_CURVE('',#5435,#5436,#2888,.T.);
#6631=EDGE_CURVE('',#5436,#5369,#2889,.T.);
#6632=EDGE_CURVE('',#5436,#5437,#2890,.T.);
#6633=EDGE_CURVE('',#5437,#5368,#2891,.T.);
#6634=EDGE_CURVE('',#5437,#5438,#2892,.T.);
#6635=EDGE_CURVE('',#5438,#5367,#2893,.T.);
#6636=EDGE_CURVE('',#5438,#5414,#2894,.T.);
#6637=EDGE_CURVE('',#5366,#5416,#4871,.T.);
#6638=EDGE_CURVE('',#5416,#5418,#4872,.T.);
#6639=EDGE_CURVE('',#5418,#5420,#4873,.T.);
#6640=EDGE_CURVE('',#5420,#5422,#4874,.T.);
#6641=EDGE_CURVE('',#5422,#5424,#4875,.T.);
#6642=EDGE_CURVE('',#5424,#5426,#4876,.T.);
#6643=EDGE_CURVE('',#5426,#5428,#4877,.T.);
#6644=EDGE_CURVE('',#5428,#5376,#4878,.T.);
#6645=EDGE_CURVE('',#5439,#5439,#4879,.T.);
#6646=EDGE_CURVE('',#5439,#5388,#2895,.T.);
#8474=ORIENTED_EDGE('',*,*,#6448,.F.);
#8475=ORIENTED_EDGE('',*,*,#6449,.F.);
#8476=ORIENTED_EDGE('',*,*,#6450,.T.);
#8477=ORIENTED_EDGE('',*,*,#6451,.F.);
#8478=ORIENTED_EDGE('',*,*,#6450,.F.);
#8479=ORIENTED_EDGE('',*,*,#6452,.F.);
#8480=ORIENTED_EDGE('',*,*,#6453,.T.);
#8481=ORIENTED_EDGE('',*,*,#6454,.F.);
#8482=ORIENTED_EDGE('',*,*,#6453,.F.);
#8483=ORIENTED_EDGE('',*,*,#6448,.T.);
#8484=ORIENTED_EDGE('',*,*,#6449,.T.);
#8485=ORIENTED_EDGE('',*,*,#6455,.F.);
#8486=ORIENTED_EDGE('',*,*,#6456,.T.);
#8487=ORIENTED_EDGE('',*,*,#6457,.F.);
#8488=ORIENTED_EDGE('',*,*,#6458,.F.);
#8489=ORIENTED_EDGE('',*,*,#6459,.F.);
#8490=ORIENTED_EDGE('',*,*,#6458,.T.);
#8491=ORIENTED_EDGE('',*,*,#6460,.F.);
#8492=ORIENTED_EDGE('',*,*,#6461,.F.);
#8493=ORIENTED_EDGE('',*,*,#6462,.F.);
#8494=ORIENTED_EDGE('',*,*,#6461,.T.);
#8495=ORIENTED_EDGE('',*,*,#6463,.F.);
#8496=ORIENTED_EDGE('',*,*,#6464,.F.);
#8497=ORIENTED_EDGE('',*,*,#6465,.F.);
#8498=ORIENTED_EDGE('',*,*,#6464,.T.);
#8499=ORIENTED_EDGE('',*,*,#6466,.F.);
#8500=ORIENTED_EDGE('',*,*,#6467,.F.);
#8501=ORIENTED_EDGE('',*,*,#6468,.F.);
#8502=ORIENTED_EDGE('',*,*,#6467,.T.);
#8503=ORIENTED_EDGE('',*,*,#6469,.F.);
#8504=ORIENTED_EDGE('',*,*,#6470,.F.);
#8505=ORIENTED_EDGE('',*,*,#6471,.F.);
#8506=ORIENTED_EDGE('',*,*,#6470,.T.);
#8507=ORIENTED_EDGE('',*,*,#6472,.F.);
#8508=ORIENTED_EDGE('',*,*,#6473,.F.);
#8509=ORIENTED_EDGE('',*,*,#6474,.F.);
#8510=ORIENTED_EDGE('',*,*,#6473,.T.);
#8511=ORIENTED_EDGE('',*,*,#6475,.F.);
#8512=ORIENTED_EDGE('',*,*,#6476,.F.);
#8513=ORIENTED_EDGE('',*,*,#6477,.F.);
#8514=ORIENTED_EDGE('',*,*,#6476,.T.);
#8515=ORIENTED_EDGE('',*,*,#6478,.F.);
#8516=ORIENTED_EDGE('',*,*,#6479,.F.);
#8517=ORIENTED_EDGE('',*,*,#6480,.F.);
#8518=ORIENTED_EDGE('',*,*,#6479,.T.);
#8519=ORIENTED_EDGE('',*,*,#6481,.F.);
#8520=ORIENTED_EDGE('',*,*,#6482,.F.);
#8521=ORIENTED_EDGE('',*,*,#6483,.F.);
#8522=ORIENTED_EDGE('',*,*,#6482,.T.);
#8523=ORIENTED_EDGE('',*,*,#6484,.F.);
#8524=ORIENTED_EDGE('',*,*,#6485,.F.);
#8525=ORIENTED_EDGE('',*,*,#6486,.F.);
#8526=ORIENTED_EDGE('',*,*,#6485,.T.);
#8527=ORIENTED_EDGE('',*,*,#6487,.F.);
#8528=ORIENTED_EDGE('',*,*,#6488,.F.);
#8529=ORIENTED_EDGE('',*,*,#6489,.F.);
#8530=ORIENTED_EDGE('',*,*,#6488,.T.);
#8531=ORIENTED_EDGE('',*,*,#6490,.F.);
#8532=ORIENTED_EDGE('',*,*,#6491,.F.);
#8533=ORIENTED_EDGE('',*,*,#6492,.F.);
#8534=ORIENTED_EDGE('',*,*,#6491,.T.);
#8535=ORIENTED_EDGE('',*,*,#6493,.F.);
#8536=ORIENTED_EDGE('',*,*,#6494,.F.);
#8537=ORIENTED_EDGE('',*,*,#6495,.F.);
#8538=ORIENTED_EDGE('',*,*,#6494,.T.);
#8539=ORIENTED_EDGE('',*,*,#6496,.F.);
#8540=ORIENTED_EDGE('',*,*,#6497,.F.);
#8541=ORIENTED_EDGE('',*,*,#6498,.F.);
#8542=ORIENTED_EDGE('',*,*,#6497,.T.);
#8543=ORIENTED_EDGE('',*,*,#6499,.F.);
#8544=ORIENTED_EDGE('',*,*,#6500,.F.);
#8545=ORIENTED_EDGE('',*,*,#6501,.F.);
#8546=ORIENTED_EDGE('',*,*,#6500,.T.);
#8547=ORIENTED_EDGE('',*,*,#6502,.F.);
#8548=ORIENTED_EDGE('',*,*,#6503,.F.);
#8549=ORIENTED_EDGE('',*,*,#6504,.F.);
#8550=ORIENTED_EDGE('',*,*,#6503,.T.);
#8551=ORIENTED_EDGE('',*,*,#6505,.F.);
#8552=ORIENTED_EDGE('',*,*,#6506,.F.);
#8553=ORIENTED_EDGE('',*,*,#6507,.F.);
#8554=ORIENTED_EDGE('',*,*,#6506,.T.);
#8555=ORIENTED_EDGE('',*,*,#6508,.F.);
#8556=ORIENTED_EDGE('',*,*,#6456,.F.);
#8557=ORIENTED_EDGE('',*,*,#6507,.T.);
#8558=ORIENTED_EDGE('',*,*,#6455,.T.);
#8559=ORIENTED_EDGE('',*,*,#6459,.T.);
#8560=ORIENTED_EDGE('',*,*,#6462,.T.);
#8561=ORIENTED_EDGE('',*,*,#6465,.T.);
#8562=ORIENTED_EDGE('',*,*,#6468,.T.);
#8563=ORIENTED_EDGE('',*,*,#6471,.T.);
#8564=ORIENTED_EDGE('',*,*,#6474,.T.);
#8565=ORIENTED_EDGE('',*,*,#6477,.T.);
#8566=ORIENTED_EDGE('',*,*,#6480,.T.);
#8567=ORIENTED_EDGE('',*,*,#6483,.T.);
#8568=ORIENTED_EDGE('',*,*,#6486,.T.);
#8569=ORIENTED_EDGE('',*,*,#6489,.T.);
#8570=ORIENTED_EDGE('',*,*,#6492,.T.);
#8571=ORIENTED_EDGE('',*,*,#6495,.T.);
#8572=ORIENTED_EDGE('',*,*,#6498,.T.);
#8573=ORIENTED_EDGE('',*,*,#6501,.T.);
#8574=ORIENTED_EDGE('',*,*,#6504,.T.);
#8575=ORIENTED_EDGE('',*,*,#6457,.T.);
#8576=ORIENTED_EDGE('',*,*,#6509,.T.);
#8577=ORIENTED_EDGE('',*,*,#6460,.T.);
#8578=ORIENTED_EDGE('',*,*,#6510,.T.);
#8579=ORIENTED_EDGE('',*,*,#6463,.T.);
#8580=ORIENTED_EDGE('',*,*,#6511,.T.);
#8581=ORIENTED_EDGE('',*,*,#6466,.T.);
#8582=ORIENTED_EDGE('',*,*,#6512,.T.);
#8583=ORIENTED_EDGE('',*,*,#6469,.T.);
#8584=ORIENTED_EDGE('',*,*,#6513,.T.);
#8585=ORIENTED_EDGE('',*,*,#6472,.T.);
#8586=ORIENTED_EDGE('',*,*,#6514,.T.);
#8587=ORIENTED_EDGE('',*,*,#6475,.T.);
#8588=ORIENTED_EDGE('',*,*,#6515,.T.);
#8589=ORIENTED_EDGE('',*,*,#6478,.T.);
#8590=ORIENTED_EDGE('',*,*,#6516,.T.);
#8591=ORIENTED_EDGE('',*,*,#6481,.T.);
#8592=ORIENTED_EDGE('',*,*,#6517,.T.);
#8593=ORIENTED_EDGE('',*,*,#6518,.T.);
#8594=ORIENTED_EDGE('',*,*,#6519,.T.);
#8595=ORIENTED_EDGE('',*,*,#6520,.T.);
#8596=ORIENTED_EDGE('',*,*,#6521,.T.);
#8597=ORIENTED_EDGE('',*,*,#6522,.T.);
#8598=ORIENTED_EDGE('',*,*,#6523,.T.);
#8599=ORIENTED_EDGE('',*,*,#6524,.T.);
#8600=ORIENTED_EDGE('',*,*,#6525,.T.);
#8601=ORIENTED_EDGE('',*,*,#6526,.T.);
#8602=ORIENTED_EDGE('',*,*,#6527,.T.);
#8603=ORIENTED_EDGE('',*,*,#6528,.T.);
#8604=ORIENTED_EDGE('',*,*,#6529,.T.);
#8605=ORIENTED_EDGE('',*,*,#6530,.T.);
#8606=ORIENTED_EDGE('',*,*,#6531,.T.);
#8607=ORIENTED_EDGE('',*,*,#6532,.T.);
#8608=ORIENTED_EDGE('',*,*,#6533,.T.);
#8609=ORIENTED_EDGE('',*,*,#6534,.T.);
#8610=ORIENTED_EDGE('',*,*,#6535,.T.);
#8611=ORIENTED_EDGE('',*,*,#6536,.T.);
#8612=ORIENTED_EDGE('',*,*,#6537,.T.);
#8613=ORIENTED_EDGE('',*,*,#6538,.T.);
#8614=ORIENTED_EDGE('',*,*,#6539,.T.);
#8615=ORIENTED_EDGE('',*,*,#6540,.T.);
#8616=ORIENTED_EDGE('',*,*,#6508,.T.);
#8617=ORIENTED_EDGE('',*,*,#6505,.T.);
#8618=ORIENTED_EDGE('',*,*,#6502,.T.);
#8619=ORIENTED_EDGE('',*,*,#6499,.T.);
#8620=ORIENTED_EDGE('',*,*,#6496,.T.);
#8621=ORIENTED_EDGE('',*,*,#6493,.T.);
#8622=ORIENTED_EDGE('',*,*,#6490,.T.);
#8623=ORIENTED_EDGE('',*,*,#6487,.T.);
#8624=ORIENTED_EDGE('',*,*,#6484,.T.);
#8625=ORIENTED_EDGE('',*,*,#6454,.T.);
#8626=ORIENTED_EDGE('',*,*,#6541,.F.);
#8627=ORIENTED_EDGE('',*,*,#6542,.T.);
#8628=ORIENTED_EDGE('',*,*,#6543,.F.);
#8629=ORIENTED_EDGE('',*,*,#6544,.F.);
#8630=ORIENTED_EDGE('',*,*,#6545,.F.);
#8631=ORIENTED_EDGE('',*,*,#6544,.T.);
#8632=ORIENTED_EDGE('',*,*,#6546,.F.);
#8633=ORIENTED_EDGE('',*,*,#6547,.F.);
#8634=ORIENTED_EDGE('',*,*,#6548,.F.);
#8635=ORIENTED_EDGE('',*,*,#6547,.T.);
#8636=ORIENTED_EDGE('',*,*,#6549,.F.);
#8637=ORIENTED_EDGE('',*,*,#6550,.F.);
#8638=ORIENTED_EDGE('',*,*,#6551,.F.);
#8639=ORIENTED_EDGE('',*,*,#6550,.T.);
#8640=ORIENTED_EDGE('',*,*,#6552,.F.);
#8641=ORIENTED_EDGE('',*,*,#6553,.F.);
#8642=ORIENTED_EDGE('',*,*,#6554,.F.);
#8643=ORIENTED_EDGE('',*,*,#6553,.T.);
#8644=ORIENTED_EDGE('',*,*,#6555,.F.);
#8645=ORIENTED_EDGE('',*,*,#6556,.F.);
#8646=ORIENTED_EDGE('',*,*,#6557,.F.);
#8647=ORIENTED_EDGE('',*,*,#6556,.T.);
#8648=ORIENTED_EDGE('',*,*,#6558,.F.);
#8649=ORIENTED_EDGE('',*,*,#6559,.F.);
#8650=ORIENTED_EDGE('',*,*,#6560,.F.);
#8651=ORIENTED_EDGE('',*,*,#6559,.T.);
#8652=ORIENTED_EDGE('',*,*,#6561,.F.);
#8653=ORIENTED_EDGE('',*,*,#6562,.F.);
#8654=ORIENTED_EDGE('',*,*,#6563,.F.);
#8655=ORIENTED_EDGE('',*,*,#6562,.T.);
#8656=ORIENTED_EDGE('',*,*,#6564,.F.);
#8657=ORIENTED_EDGE('',*,*,#6565,.F.);
#8658=ORIENTED_EDGE('',*,*,#6566,.F.);
#8659=ORIENTED_EDGE('',*,*,#6565,.T.);
#8660=ORIENTED_EDGE('',*,*,#6538,.F.);
#8661=ORIENTED_EDGE('',*,*,#6567,.F.);
#8662=ORIENTED_EDGE('',*,*,#6568,.F.);
#8663=ORIENTED_EDGE('',*,*,#6567,.T.);
#8664=ORIENTED_EDGE('',*,*,#6537,.F.);
#8665=ORIENTED_EDGE('',*,*,#6569,.F.);
#8666=ORIENTED_EDGE('',*,*,#6570,.F.);
#8667=ORIENTED_EDGE('',*,*,#6569,.T.);
#8668=ORIENTED_EDGE('',*,*,#6536,.F.);
#8669=ORIENTED_EDGE('',*,*,#6571,.F.);
#8670=ORIENTED_EDGE('',*,*,#6572,.F.);
#8671=ORIENTED_EDGE('',*,*,#6571,.T.);
#8672=ORIENTED_EDGE('',*,*,#6535,.F.);
#8673=ORIENTED_EDGE('',*,*,#6573,.F.);
#8674=ORIENTED_EDGE('',*,*,#6574,.F.);
#8675=ORIENTED_EDGE('',*,*,#6573,.T.);
#8676=ORIENTED_EDGE('',*,*,#6534,.F.);
#8677=ORIENTED_EDGE('',*,*,#6575,.F.);
#8678=ORIENTED_EDGE('',*,*,#6576,.F.);
#8679=ORIENTED_EDGE('',*,*,#6575,.T.);
#8680=ORIENTED_EDGE('',*,*,#6533,.F.);
#8681=ORIENTED_EDGE('',*,*,#6577,.F.);
#8682=ORIENTED_EDGE('',*,*,#6578,.F.);
#8683=ORIENTED_EDGE('',*,*,#6577,.T.);
#8684=ORIENTED_EDGE('',*,*,#6532,.F.);
#8685=ORIENTED_EDGE('',*,*,#6579,.F.);
#8686=ORIENTED_EDGE('',*,*,#6580,.F.);
#8687=ORIENTED_EDGE('',*,*,#6579,.T.);
#8688=ORIENTED_EDGE('',*,*,#6531,.F.);
#8689=ORIENTED_EDGE('',*,*,#6581,.F.);
#8690=ORIENTED_EDGE('',*,*,#6582,.F.);
#8691=ORIENTED_EDGE('',*,*,#6581,.T.);
#8692=ORIENTED_EDGE('',*,*,#6530,.F.);
#8693=ORIENTED_EDGE('',*,*,#6583,.F.);
#8694=ORIENTED_EDGE('',*,*,#6584,.F.);
#8695=ORIENTED_EDGE('',*,*,#6583,.T.);
#8696=ORIENTED_EDGE('',*,*,#6529,.F.);
#8697=ORIENTED_EDGE('',*,*,#6542,.F.);
#8698=ORIENTED_EDGE('',*,*,#6584,.T.);
#8699=ORIENTED_EDGE('',*,*,#6541,.T.);
#8700=ORIENTED_EDGE('',*,*,#6545,.T.);
#8701=ORIENTED_EDGE('',*,*,#6548,.T.);
#8702=ORIENTED_EDGE('',*,*,#6551,.T.);
#8703=ORIENTED_EDGE('',*,*,#6554,.T.);
#8704=ORIENTED_EDGE('',*,*,#6557,.T.);
#8705=ORIENTED_EDGE('',*,*,#6560,.T.);
#8706=ORIENTED_EDGE('',*,*,#6563,.T.);
#8707=ORIENTED_EDGE('',*,*,#6566,.T.);
#8708=ORIENTED_EDGE('',*,*,#6568,.T.);
#8709=ORIENTED_EDGE('',*,*,#6570,.T.);
#8710=ORIENTED_EDGE('',*,*,#6572,.T.);
#8711=ORIENTED_EDGE('',*,*,#6574,.T.);
#8712=ORIENTED_EDGE('',*,*,#6576,.T.);
#8713=ORIENTED_EDGE('',*,*,#6578,.T.);
#8714=ORIENTED_EDGE('',*,*,#6580,.T.);
#8715=ORIENTED_EDGE('',*,*,#6582,.T.);
#8716=ORIENTED_EDGE('',*,*,#6543,.T.);
#8717=ORIENTED_EDGE('',*,*,#6585,.T.);
#8718=ORIENTED_EDGE('',*,*,#6546,.T.);
#8719=ORIENTED_EDGE('',*,*,#6586,.T.);
#8720=ORIENTED_EDGE('',*,*,#6549,.T.);
#8721=ORIENTED_EDGE('',*,*,#6587,.T.);
#8722=ORIENTED_EDGE('',*,*,#6552,.T.);
#8723=ORIENTED_EDGE('',*,*,#6588,.T.);
#8724=ORIENTED_EDGE('',*,*,#6555,.T.);
#8725=ORIENTED_EDGE('',*,*,#6589,.T.);
#8726=ORIENTED_EDGE('',*,*,#6558,.T.);
#8727=ORIENTED_EDGE('',*,*,#6590,.T.);
#8728=ORIENTED_EDGE('',*,*,#6561,.T.);
#8729=ORIENTED_EDGE('',*,*,#6591,.T.);
#8730=ORIENTED_EDGE('',*,*,#6564,.T.);
#8731=ORIENTED_EDGE('',*,*,#6592,.T.);
#8732=ORIENTED_EDGE('',*,*,#6593,.F.);
#8733=ORIENTED_EDGE('',*,*,#6594,.T.);
#8734=ORIENTED_EDGE('',*,*,#6595,.F.);
#8735=ORIENTED_EDGE('',*,*,#6596,.F.);
#8736=ORIENTED_EDGE('',*,*,#6597,.F.);
#8737=ORIENTED_EDGE('',*,*,#6596,.T.);
#8738=ORIENTED_EDGE('',*,*,#6598,.F.);
#8739=ORIENTED_EDGE('',*,*,#6599,.F.);
#8740=ORIENTED_EDGE('',*,*,#6600,.F.);
#8741=ORIENTED_EDGE('',*,*,#6599,.T.);
#8742=ORIENTED_EDGE('',*,*,#6601,.F.);
#8743=ORIENTED_EDGE('',*,*,#6602,.F.);
#8744=ORIENTED_EDGE('',*,*,#6603,.F.);
#8745=ORIENTED_EDGE('',*,*,#6602,.T.);
#8746=ORIENTED_EDGE('',*,*,#6604,.F.);
#8747=ORIENTED_EDGE('',*,*,#6605,.F.);
#8748=ORIENTED_EDGE('',*,*,#6606,.F.);
#8749=ORIENTED_EDGE('',*,*,#6605,.T.);
#8750=ORIENTED_EDGE('',*,*,#6607,.F.);
#8751=ORIENTED_EDGE('',*,*,#6608,.F.);
#8752=ORIENTED_EDGE('',*,*,#6609,.F.);
#8753=ORIENTED_EDGE('',*,*,#6608,.T.);
#8754=ORIENTED_EDGE('',*,*,#6610,.F.);
#8755=ORIENTED_EDGE('',*,*,#6611,.F.);
#8756=ORIENTED_EDGE('',*,*,#6612,.F.);
#8757=ORIENTED_EDGE('',*,*,#6611,.T.);
#8758=ORIENTED_EDGE('',*,*,#6613,.F.);
#8759=ORIENTED_EDGE('',*,*,#6614,.F.);
#8760=ORIENTED_EDGE('',*,*,#6615,.F.);
#8761=ORIENTED_EDGE('',*,*,#6614,.T.);
#8762=ORIENTED_EDGE('',*,*,#6616,.F.);
#8763=ORIENTED_EDGE('',*,*,#6617,.F.);
#8764=ORIENTED_EDGE('',*,*,#6618,.F.);
#8765=ORIENTED_EDGE('',*,*,#6617,.T.);
#8766=ORIENTED_EDGE('',*,*,#6527,.F.);
#8767=ORIENTED_EDGE('',*,*,#6619,.F.);
#8768=ORIENTED_EDGE('',*,*,#6620,.F.);
#8769=ORIENTED_EDGE('',*,*,#6619,.T.);
#8770=ORIENTED_EDGE('',*,*,#6526,.F.);
#8771=ORIENTED_EDGE('',*,*,#6621,.F.);
#8772=ORIENTED_EDGE('',*,*,#6622,.F.);
#8773=ORIENTED_EDGE('',*,*,#6621,.T.);
#8774=ORIENTED_EDGE('',*,*,#6525,.F.);
#8775=ORIENTED_EDGE('',*,*,#6623,.F.);
#8776=ORIENTED_EDGE('',*,*,#6624,.F.);
#8777=ORIENTED_EDGE('',*,*,#6623,.T.);
#8778=ORIENTED_EDGE('',*,*,#6524,.F.);
#8779=ORIENTED_EDGE('',*,*,#6625,.F.);
#8780=ORIENTED_EDGE('',*,*,#6626,.F.);
#8781=ORIENTED_EDGE('',*,*,#6625,.T.);
#8782=ORIENTED_EDGE('',*,*,#6523,.F.);
#8783=ORIENTED_EDGE('',*,*,#6627,.F.);
#8784=ORIENTED_EDGE('',*,*,#6628,.F.);
#8785=ORIENTED_EDGE('',*,*,#6627,.T.);
#8786=ORIENTED_EDGE('',*,*,#6522,.F.);
#8787=ORIENTED_EDGE('',*,*,#6629,.F.);
#8788=ORIENTED_EDGE('',*,*,#6630,.F.);
#8789=ORIENTED_EDGE('',*,*,#6629,.T.);
#8790=ORIENTED_EDGE('',*,*,#6521,.F.);
#8791=ORIENTED_EDGE('',*,*,#6631,.F.);
#8792=ORIENTED_EDGE('',*,*,#6632,.F.);
#8793=ORIENTED_EDGE('',*,*,#6631,.T.);
#8794=ORIENTED_EDGE('',*,*,#6520,.F.);
#8795=ORIENTED_EDGE('',*,*,#6633,.F.);
#8796=ORIENTED_EDGE('',*,*,#6634,.F.);
#8797=ORIENTED_EDGE('',*,*,#6633,.T.);
#8798=ORIENTED_EDGE('',*,*,#6519,.F.);
#8799=ORIENTED_EDGE('',*,*,#6635,.F.);
#8800=ORIENTED_EDGE('',*,*,#6636,.F.);
#8801=ORIENTED_EDGE('',*,*,#6635,.T.);
#8802=ORIENTED_EDGE('',*,*,#6518,.F.);
#8803=ORIENTED_EDGE('',*,*,#6594,.F.);
#8804=ORIENTED_EDGE('',*,*,#6636,.T.);
#8805=ORIENTED_EDGE('',*,*,#6593,.T.);
#8806=ORIENTED_EDGE('',*,*,#6597,.T.);
#8807=ORIENTED_EDGE('',*,*,#6600,.T.);
#8808=ORIENTED_EDGE('',*,*,#6603,.T.);
#8809=ORIENTED_EDGE('',*,*,#6606,.T.);
#8810=ORIENTED_EDGE('',*,*,#6609,.T.);
#8811=ORIENTED_EDGE('',*,*,#6612,.T.);
#8812=ORIENTED_EDGE('',*,*,#6615,.T.);
#8813=ORIENTED_EDGE('',*,*,#6618,.T.);
#8814=ORIENTED_EDGE('',*,*,#6620,.T.);
#8815=ORIENTED_EDGE('',*,*,#6622,.T.);
#8816=ORIENTED_EDGE('',*,*,#6624,.T.);
#8817=ORIENTED_EDGE('',*,*,#6626,.T.);
#8818=ORIENTED_EDGE('',*,*,#6628,.T.);
#8819=ORIENTED_EDGE('',*,*,#6630,.T.);
#8820=ORIENTED_EDGE('',*,*,#6632,.T.);
#8821=ORIENTED_EDGE('',*,*,#6634,.T.);
#8822=ORIENTED_EDGE('',*,*,#6595,.T.);
#8823=ORIENTED_EDGE('',*,*,#6637,.T.);
#8824=ORIENTED_EDGE('',*,*,#6598,.T.);
#8825=ORIENTED_EDGE('',*,*,#6638,.T.);
#8826=ORIENTED_EDGE('',*,*,#6601,.T.);
#8827=ORIENTED_EDGE('',*,*,#6639,.T.);
#8828=ORIENTED_EDGE('',*,*,#6604,.T.);
#8829=ORIENTED_EDGE('',*,*,#6640,.T.);
#8830=ORIENTED_EDGE('',*,*,#6607,.T.);
#8831=ORIENTED_EDGE('',*,*,#6641,.T.);
#8832=ORIENTED_EDGE('',*,*,#6610,.T.);
#8833=ORIENTED_EDGE('',*,*,#6642,.T.);
#8834=ORIENTED_EDGE('',*,*,#6613,.T.);
#8835=ORIENTED_EDGE('',*,*,#6643,.T.);
#8836=ORIENTED_EDGE('',*,*,#6616,.T.);
#8837=ORIENTED_EDGE('',*,*,#6644,.T.);
#8838=ORIENTED_EDGE('',*,*,#6645,.F.);
#8839=ORIENTED_EDGE('',*,*,#6646,.T.);
#8840=ORIENTED_EDGE('',*,*,#6539,.F.);
#8841=ORIENTED_EDGE('',*,*,#6592,.F.);
#8842=ORIENTED_EDGE('',*,*,#6591,.F.);
#8843=ORIENTED_EDGE('',*,*,#6590,.F.);
#8844=ORIENTED_EDGE('',*,*,#6589,.F.);
#8845=ORIENTED_EDGE('',*,*,#6588,.F.);
#8846=ORIENTED_EDGE('',*,*,#6587,.F.);
#8847=ORIENTED_EDGE('',*,*,#6586,.F.);
#8848=ORIENTED_EDGE('',*,*,#6585,.F.);
#8849=ORIENTED_EDGE('',*,*,#6528,.F.);
#8850=ORIENTED_EDGE('',*,*,#6644,.F.);
#8851=ORIENTED_EDGE('',*,*,#6643,.F.);
#8852=ORIENTED_EDGE('',*,*,#6642,.F.);
#8853=ORIENTED_EDGE('',*,*,#6641,.F.);
#8854=ORIENTED_EDGE('',*,*,#6640,.F.);
#8855=ORIENTED_EDGE('',*,*,#6639,.F.);
#8856=ORIENTED_EDGE('',*,*,#6638,.F.);
#8857=ORIENTED_EDGE('',*,*,#6637,.F.);
#8858=ORIENTED_EDGE('',*,*,#6517,.F.);
#8859=ORIENTED_EDGE('',*,*,#6516,.F.);
#8860=ORIENTED_EDGE('',*,*,#6515,.F.);
#8861=ORIENTED_EDGE('',*,*,#6514,.F.);
#8862=ORIENTED_EDGE('',*,*,#6513,.F.);
#8863=ORIENTED_EDGE('',*,*,#6512,.F.);
#8864=ORIENTED_EDGE('',*,*,#6511,.F.);
#8865=ORIENTED_EDGE('',*,*,#6510,.F.);
#8866=ORIENTED_EDGE('',*,*,#6509,.F.);
#8867=ORIENTED_EDGE('',*,*,#6540,.F.);
#8868=ORIENTED_EDGE('',*,*,#6646,.F.);
#8869=ORIENTED_EDGE('',*,*,#6451,.T.);
#8870=ORIENTED_EDGE('',*,*,#6645,.T.);
#8871=ORIENTED_EDGE('',*,*,#6452,.T.);
#10347=CYLINDRICAL_SURFACE('',#11865,0.21);
#10348=CYLINDRICAL_SURFACE('',#11866,0.6);
#10349=CYLINDRICAL_SURFACE('',#11979,1.37);
#10629=ADVANCED_FACE('',(#1287),#10347,.F.);
#10630=ADVANCED_FACE('',(#1288,#506),#10348,.F.);
#10631=ADVANCED_FACE('',(#1289),#694,.T.);
#10632=ADVANCED_FACE('',(#1290),#695,.T.);
#10633=ADVANCED_FACE('',(#1291),#696,.T.);
#10634=ADVANCED_FACE('',(#1292),#697,.T.);
#10635=ADVANCED_FACE('',(#1293),#698,.T.);
#10636=ADVANCED_FACE('',(#1294),#699,.T.);
#10637=ADVANCED_FACE('',(#1295),#700,.T.);
#10638=ADVANCED_FACE('',(#1296),#701,.T.);
#10639=ADVANCED_FACE('',(#1297),#702,.T.);
#10640=ADVANCED_FACE('',(#1298),#703,.T.);
#10641=ADVANCED_FACE('',(#1299),#704,.T.);
#10642=ADVANCED_FACE('',(#1300),#705,.T.);
#10643=ADVANCED_FACE('',(#1301),#706,.T.);
#10644=ADVANCED_FACE('',(#1302),#707,.T.);
#10645=ADVANCED_FACE('',(#1303),#708,.T.);
#10646=ADVANCED_FACE('',(#1304),#709,.T.);
#10647=ADVANCED_FACE('',(#1305),#710,.T.);
#10648=ADVANCED_FACE('',(#1306),#711,.T.);
#10649=ADVANCED_FACE('',(#1307),#712,.T.);
#10650=ADVANCED_FACE('',(#1308),#713,.T.);
#10651=ADVANCED_FACE('',(#1309),#714,.T.);
#10652=ADVANCED_FACE('',(#1310),#715,.T.);
#10653=ADVANCED_FACE('',(#1311),#716,.T.);
#10654=ADVANCED_FACE('',(#1312),#717,.T.);
#10655=ADVANCED_FACE('',(#1313),#718,.T.);
#10656=ADVANCED_FACE('',(#1314),#719,.T.);
#10657=ADVANCED_FACE('',(#1315),#720,.T.);
#10658=ADVANCED_FACE('',(#1316,#507),#721,.T.);
#10659=ADVANCED_FACE('',(#1317),#722,.T.);
#10660=ADVANCED_FACE('',(#1318),#723,.T.);
#10661=ADVANCED_FACE('',(#1319),#724,.T.);
#10662=ADVANCED_FACE('',(#1320),#725,.T.);
#10663=ADVANCED_FACE('',(#1321),#726,.T.);
#10664=ADVANCED_FACE('',(#1322),#727,.T.);
#10665=ADVANCED_FACE('',(#1323),#728,.T.);
#10666=ADVANCED_FACE('',(#1324),#729,.T.);
#10667=ADVANCED_FACE('',(#1325),#730,.T.);
#10668=ADVANCED_FACE('',(#1326),#731,.T.);
#10669=ADVANCED_FACE('',(#1327),#732,.T.);
#10670=ADVANCED_FACE('',(#1328),#733,.T.);
#10671=ADVANCED_FACE('',(#1329),#734,.T.);
#10672=ADVANCED_FACE('',(#1330),#735,.T.);
#10673=ADVANCED_FACE('',(#1331),#736,.T.);
#10674=ADVANCED_FACE('',(#1332),#737,.T.);
#10675=ADVANCED_FACE('',(#1333),#738,.T.);
#10676=ADVANCED_FACE('',(#1334),#739,.T.);
#10677=ADVANCED_FACE('',(#1335),#740,.T.);
#10678=ADVANCED_FACE('',(#1336),#741,.T.);
#10679=ADVANCED_FACE('',(#1337),#742,.T.);
#10680=ADVANCED_FACE('',(#1338),#743,.T.);
#10681=ADVANCED_FACE('',(#1339),#744,.T.);
#10682=ADVANCED_FACE('',(#1340),#745,.T.);
#10683=ADVANCED_FACE('',(#1341),#746,.T.);
#10684=ADVANCED_FACE('',(#1342),#747,.T.);
#10685=ADVANCED_FACE('',(#1343),#748,.T.);
#10686=ADVANCED_FACE('',(#1344),#749,.T.);
#10687=ADVANCED_FACE('',(#1345),#750,.T.);
#10688=ADVANCED_FACE('',(#1346),#751,.T.);
#10689=ADVANCED_FACE('',(#1347),#752,.T.);
#10690=ADVANCED_FACE('',(#1348),#753,.T.);
#10691=ADVANCED_FACE('',(#1349),#754,.T.);
#10692=ADVANCED_FACE('',(#1350),#755,.T.);
#10693=ADVANCED_FACE('',(#1351),#756,.T.);
#10694=ADVANCED_FACE('',(#1352),#757,.T.);
#10695=ADVANCED_FACE('',(#1353),#758,.T.);
#10696=ADVANCED_FACE('',(#1354),#759,.T.);
#10697=ADVANCED_FACE('',(#1355),#760,.T.);
#10698=ADVANCED_FACE('',(#1356),#761,.T.);
#10699=ADVANCED_FACE('',(#1357),#762,.T.);
#10700=ADVANCED_FACE('',(#1358),#763,.T.);
#10701=ADVANCED_FACE('',(#1359),#764,.T.);
#10702=ADVANCED_FACE('',(#1360),#765,.T.);
#10703=ADVANCED_FACE('',(#1361),#766,.T.);
#10704=ADVANCED_FACE('',(#1362),#767,.T.);
#10705=ADVANCED_FACE('',(#1363),#768,.T.);
#10706=ADVANCED_FACE('',(#1364),#769,.T.);
#10707=ADVANCED_FACE('',(#1365),#770,.T.);
#10708=ADVANCED_FACE('',(#1366),#771,.T.);
#10709=ADVANCED_FACE('',(#1367),#772,.T.);
#10710=ADVANCED_FACE('',(#1368),#773,.T.);
#10711=ADVANCED_FACE('',(#1369),#774,.T.);
#10712=ADVANCED_FACE('',(#1370),#775,.T.);
#10713=ADVANCED_FACE('',(#1371,#508),#10349,.T.);
#10714=ADVANCED_FACE('',(#1372,#509),#776,.F.);
#11013=CLOSED_SHELL('',(#10629,#10630,#10631,#10632,#10633,#10634,#10635,
#10636,#10637,#10638,#10639,#10640,#10641,#10642,#10643,#10644,#10645,#10646,
#10647,#10648,#10649,#10650,#10651,#10652,#10653,#10654,#10655,#10656,#10657,
#10658,#10659,#10660,#10661,#10662,#10663,#10664,#10665,#10666,#10667,#10668,
#10669,#10670,#10671,#10672,#10673,#10674,#10675,#10676,#10677,#10678,#10679,
#10680,#10681,#10682,#10683,#10684,#10685,#10686,#10687,#10688,#10689,#10690,
#10691,#10692,#10693,#10694,#10695,#10696,#10697,#10698,#10699,#10700,#10701,
#10702,#10703,#10704,#10705,#10706,#10707,#10708,#10709,#10710,#10711,#10712,
#10713,#10714));
#11864=AXIS2_PLACEMENT_3D('',#17312,#13678,#13679);
#11865=AXIS2_PLACEMENT_3D('',#17313,#13680,#13681);
#11866=AXIS2_PLACEMENT_3D('',#17388,#13683,#13684);
#11867=AXIS2_PLACEMENT_3D('',#17390,#13685,#13686);
#11868=AXIS2_PLACEMENT_3D('',#17393,#13688,#13689);
#11869=AXIS2_PLACEMENT_3D('',#17394,#13690,#13691);
#11870=AXIS2_PLACEMENT_3D('',#17403,#13696,#13697);
#11871=AXIS2_PLACEMENT_3D('',#17409,#13701,#13702);
#11872=AXIS2_PLACEMENT_3D('',#17415,#13706,#13707);
#11873=AXIS2_PLACEMENT_3D('',#17421,#13711,#13712);
#11874=AXIS2_PLACEMENT_3D('',#17427,#13716,#13717);
#11875=AXIS2_PLACEMENT_3D('',#17433,#13721,#13722);
#11876=AXIS2_PLACEMENT_3D('',#17439,#13726,#13727);
#11877=AXIS2_PLACEMENT_3D('',#17445,#13731,#13732);
#11878=AXIS2_PLACEMENT_3D('',#17451,#13736,#13737);
#11879=AXIS2_PLACEMENT_3D('',#17457,#13741,#13742);
#11880=AXIS2_PLACEMENT_3D('',#17463,#13746,#13747);
#11881=AXIS2_PLACEMENT_3D('',#17469,#13751,#13752);
#11882=AXIS2_PLACEMENT_3D('',#17475,#13756,#13757);
#11883=AXIS2_PLACEMENT_3D('',#17481,#13761,#13762);
#11884=AXIS2_PLACEMENT_3D('',#17487,#13766,#13767);
#11885=AXIS2_PLACEMENT_3D('',#17493,#13771,#13772);
#11886=AXIS2_PLACEMENT_3D('',#17499,#13776,#13777);
#11887=AXIS2_PLACEMENT_3D('',#17502,#13780,#13781);
#11888=AXIS2_PLACEMENT_3D('',#17503,#13782,#13783);
#11889=AXIS2_PLACEMENT_3D('',#17504,#13784,#13785);
#11890=AXIS2_PLACEMENT_3D('',#17505,#13786,#13787);
#11891=AXIS2_PLACEMENT_3D('',#17506,#13788,#13789);
#11892=AXIS2_PLACEMENT_3D('',#17507,#13790,#13791);
#11893=AXIS2_PLACEMENT_3D('',#17508,#13792,#13793);
#11894=AXIS2_PLACEMENT_3D('',#17509,#13794,#13795);
#11895=AXIS2_PLACEMENT_3D('',#17510,#13796,#13797);
#11896=AXIS2_PLACEMENT_3D('',#17511,#13798,#13799);
#11897=AXIS2_PLACEMENT_3D('',#17512,#13800,#13801);
#11898=AXIS2_PLACEMENT_3D('',#17513,#13802,#13803);
#11899=AXIS2_PLACEMENT_3D('',#17514,#13804,#13805);
#11900=AXIS2_PLACEMENT_3D('',#17515,#13806,#13807);
#11901=AXIS2_PLACEMENT_3D('',#17516,#13808,#13809);
#11902=AXIS2_PLACEMENT_3D('',#17517,#13810,#13811);
#11903=AXIS2_PLACEMENT_3D('',#17518,#13812,#13813);
#11904=AXIS2_PLACEMENT_3D('',#17519,#13814,#13815);
#11905=AXIS2_PLACEMENT_3D('',#17521,#13816,#13817);
#11906=AXIS2_PLACEMENT_3D('',#17543,#13828,#13829);
#11907=AXIS2_PLACEMENT_3D('',#17565,#13840,#13841);
#11908=AXIS2_PLACEMENT_3D('',#17566,#13842,#13843);
#11909=AXIS2_PLACEMENT_3D('',#17567,#13844,#13845);
#11910=AXIS2_PLACEMENT_3D('',#17575,#13850,#13851);
#11911=AXIS2_PLACEMENT_3D('',#17581,#13855,#13856);
#11912=AXIS2_PLACEMENT_3D('',#17587,#13860,#13861);
#11913=AXIS2_PLACEMENT_3D('',#17593,#13865,#13866);
#11914=AXIS2_PLACEMENT_3D('',#17599,#13870,#13871);
#11915=AXIS2_PLACEMENT_3D('',#17605,#13875,#13876);
#11916=AXIS2_PLACEMENT_3D('',#17611,#13880,#13881);
#11917=AXIS2_PLACEMENT_3D('',#17616,#13885,#13886);
#11918=AXIS2_PLACEMENT_3D('',#17620,#13889,#13890);
#11919=AXIS2_PLACEMENT_3D('',#17624,#13893,#13894);
#11920=AXIS2_PLACEMENT_3D('',#17628,#13897,#13898);
#11921=AXIS2_PLACEMENT_3D('',#17632,#13901,#13902);
#11922=AXIS2_PLACEMENT_3D('',#17636,#13905,#13906);
#11923=AXIS2_PLACEMENT_3D('',#17640,#13909,#13910);
#11924=AXIS2_PLACEMENT_3D('',#17644,#13913,#13914);
#11925=AXIS2_PLACEMENT_3D('',#17648,#13917,#13918);
#11926=AXIS2_PLACEMENT_3D('',#17652,#13921,#13922);
#11927=AXIS2_PLACEMENT_3D('',#17654,#13924,#13925);
#11928=AXIS2_PLACEMENT_3D('',#17655,#13926,#13927);
#11929=AXIS2_PLACEMENT_3D('',#17656,#13928,#13929);
#11930=AXIS2_PLACEMENT_3D('',#17657,#13930,#13931);
#11931=AXIS2_PLACEMENT_3D('',#17658,#13932,#13933);
#11932=AXIS2_PLACEMENT_3D('',#17659,#13934,#13935);
#11933=AXIS2_PLACEMENT_3D('',#17660,#13936,#13937);
#11934=AXIS2_PLACEMENT_3D('',#17661,#13938,#13939);
#11935=AXIS2_PLACEMENT_3D('',#17662,#13940,#13941);
#11936=AXIS2_PLACEMENT_3D('',#17663,#13942,#13943);
#11937=AXIS2_PLACEMENT_3D('',#17664,#13944,#13945);
#11938=AXIS2_PLACEMENT_3D('',#17665,#13946,#13947);
#11939=AXIS2_PLACEMENT_3D('',#17666,#13948,#13949);
#11940=AXIS2_PLACEMENT_3D('',#17667,#13950,#13951);
#11941=AXIS2_PLACEMENT_3D('',#17668,#13952,#13953);
#11942=AXIS2_PLACEMENT_3D('',#17669,#13954,#13955);
#11943=AXIS2_PLACEMENT_3D('',#17670,#13956,#13957);
#11944=AXIS2_PLACEMENT_3D('',#17671,#13958,#13959);
#11945=AXIS2_PLACEMENT_3D('',#17679,#13964,#13965);
#11946=AXIS2_PLACEMENT_3D('',#17685,#13969,#13970);
#11947=AXIS2_PLACEMENT_3D('',#17691,#13974,#13975);
#11948=AXIS2_PLACEMENT_3D('',#17697,#13979,#13980);
#11949=AXIS2_PLACEMENT_3D('',#17703,#13984,#13985);
#11950=AXIS2_PLACEMENT_3D('',#17709,#13989,#13990);
#11951=AXIS2_PLACEMENT_3D('',#17715,#13994,#13995);
#11952=AXIS2_PLACEMENT_3D('',#17720,#13999,#14000);
#11953=AXIS2_PLACEMENT_3D('',#17724,#14003,#14004);
#11954=AXIS2_PLACEMENT_3D('',#17728,#14007,#14008);
#11955=AXIS2_PLACEMENT_3D('',#17732,#14011,#14012);
#11956=AXIS2_PLACEMENT_3D('',#17736,#14015,#14016);
#11957=AXIS2_PLACEMENT_3D('',#17740,#14019,#14020);
#11958=AXIS2_PLACEMENT_3D('',#17744,#14023,#14024);
#11959=AXIS2_PLACEMENT_3D('',#17748,#14027,#14028);
#11960=AXIS2_PLACEMENT_3D('',#17752,#14031,#14032);
#11961=AXIS2_PLACEMENT_3D('',#17756,#14035,#14036);
#11962=AXIS2_PLACEMENT_3D('',#17758,#14038,#14039);
#11963=AXIS2_PLACEMENT_3D('',#17759,#14040,#14041);
#11964=AXIS2_PLACEMENT_3D('',#17760,#14042,#14043);
#11965=AXIS2_PLACEMENT_3D('',#17761,#14044,#14045);
#11966=AXIS2_PLACEMENT_3D('',#17762,#14046,#14047);
#11967=AXIS2_PLACEMENT_3D('',#17763,#14048,#14049);
#11968=AXIS2_PLACEMENT_3D('',#17764,#14050,#14051);
#11969=AXIS2_PLACEMENT_3D('',#17765,#14052,#14053);
#11970=AXIS2_PLACEMENT_3D('',#17766,#14054,#14055);
#11971=AXIS2_PLACEMENT_3D('',#17767,#14056,#14057);
#11972=AXIS2_PLACEMENT_3D('',#17768,#14058,#14059);
#11973=AXIS2_PLACEMENT_3D('',#17769,#14060,#14061);
#11974=AXIS2_PLACEMENT_3D('',#17770,#14062,#14063);
#11975=AXIS2_PLACEMENT_3D('',#17771,#14064,#14065);
#11976=AXIS2_PLACEMENT_3D('',#17772,#14066,#14067);
#11977=AXIS2_PLACEMENT_3D('',#17773,#14068,#14069);
#11978=AXIS2_PLACEMENT_3D('',#17774,#14070,#14071);
#11979=AXIS2_PLACEMENT_3D('',#17775,#14072,#14073);
#11980=AXIS2_PLACEMENT_3D('',#17777,#14074,#14075);
#11981=AXIS2_PLACEMENT_3D('',#17779,#14077,#14078);
#13678=DIRECTION('axis',(0.,0.,1.));
#13679=DIRECTION('refdir',(1.,0.,0.));
#13680=DIRECTION('center_axis',(0.,0.,1.));
#13681=DIRECTION('ref_axis',(1.,0.,0.));
#13682=DIRECTION('',(0.,0.,1.));
#13683=DIRECTION('center_axis',(0.,1.,0.));
#13684=DIRECTION('ref_axis',(1.,0.,0.));
#13685=DIRECTION('center_axis',(0.,1.,0.));
#13686=DIRECTION('ref_axis',(1.,0.,0.));
#13687=DIRECTION('',(0.,1.,0.));
#13688=DIRECTION('center_axis',(0.,-1.,0.));
#13689=DIRECTION('ref_axis',(1.,0.,0.));
#13690=DIRECTION('center_axis',(-0.762527203906389,0.,0.646956152534856));
#13691=DIRECTION('ref_axis',(-0.646956152534856,0.,-0.762527203906389));
#13692=DIRECTION('',(0.646956152534856,0.,0.762527203906389));
#13693=DIRECTION('',(0.,-1.,0.));
#13694=DIRECTION('',(-0.646956152534856,0.,-0.762527203906389));
#13695=DIRECTION('',(0.,-1.,0.));
#13696=DIRECTION('center_axis',(-0.695442635009613,0.,0.718581617779697));
#13697=DIRECTION('ref_axis',(-0.718581617779697,0.,-0.695442635009613));
#13698=DIRECTION('',(0.718581617779697,0.,0.695442635009613));
#13699=DIRECTION('',(-0.718581617779697,0.,-0.695442635009613));
#13700=DIRECTION('',(0.,-1.,0.));
#13701=DIRECTION('center_axis',(-0.621660573370079,0.,0.783286749228649));
#13702=DIRECTION('ref_axis',(-0.783286749228649,0.,-0.621660573370079));
#13703=DIRECTION('',(0.783286749228649,0.,0.621660573370079));
#13704=DIRECTION('',(-0.783286749228649,0.,-0.621660573370079));
#13705=DIRECTION('',(0.,-1.,0.));
#13706=DIRECTION('center_axis',(-0.541891580574751,0.,0.840448401094439));
#13707=DIRECTION('ref_axis',(-0.840448401094439,0.,-0.541891580574751));
#13708=DIRECTION('',(0.840448401094439,0.,0.541891580574751));
#13709=DIRECTION('',(-0.840448401094439,0.,-0.541891580574751));
#13710=DIRECTION('',(0.,-1.,0.));
#13711=DIRECTION('center_axis',(-0.456903875630423,0.,0.889516075421855));
#13712=DIRECTION('ref_axis',(-0.889516075421855,0.,-0.456903875630423));
#13713=DIRECTION('',(0.889516075421855,0.,0.456903875630423));
#13714=DIRECTION('',(-0.889516075421855,0.,-0.456903875630423));
#13715=DIRECTION('',(0.,-1.,0.));
#13716=DIRECTION('center_axis',(-0.367515936594703,0.,0.930017223684012));
#13717=DIRECTION('ref_axis',(-0.930017223684012,0.,-0.367515936594703));
#13718=DIRECTION('',(0.930017223684012,0.,0.367515936594703));
#13719=DIRECTION('',(-0.930017223684012,0.,-0.367515936594703));
#13720=DIRECTION('',(0.,-1.,0.));
#13721=DIRECTION('center_axis',(-0.274588618184932,0.,0.961561797682962));
#13722=DIRECTION('ref_axis',(-0.961561797682962,0.,-0.274588618184932));
#13723=DIRECTION('',(0.961561797682962,0.,0.274588618184932));
#13724=DIRECTION('',(-0.961561797682962,0.,-0.274588618184932));
#13725=DIRECTION('',(0.,-1.,0.));
#13726=DIRECTION('center_axis',(-0.179016861276632,0.,0.983846005927077));
#13727=DIRECTION('ref_axis',(-0.983846005927077,0.,-0.179016861276632));
#13728=DIRECTION('',(0.983846005927077,0.,0.179016861276632));
#13729=DIRECTION('',(-0.983846005927077,0.,-0.179016861276632));
#13730=DIRECTION('',(0.,-1.,0.));
#13731=DIRECTION('center_axis',(0.99144486137381,0.,0.130526192220052));
#13732=DIRECTION('ref_axis',(-0.130526192220052,0.,0.99144486137381));
#13733=DIRECTION('',(0.130526192220052,0.,-0.99144486137381));
#13734=DIRECTION('',(-0.130526192220052,0.,0.99144486137381));
#13735=DIRECTION('',(0.,-1.,0.));
#13736=DIRECTION('center_axis',(0.179016861276633,0.,-0.983846005927077));
#13737=DIRECTION('ref_axis',(0.983846005927077,0.,0.179016861276633));
#13738=DIRECTION('',(-0.983846005927077,0.,-0.179016861276633));
#13739=DIRECTION('',(0.983846005927077,0.,0.179016861276633));
#13740=DIRECTION('',(0.,-1.,0.));
#13741=DIRECTION('center_axis',(0.274588618184932,0.,-0.961561797682962));
#13742=DIRECTION('ref_axis',(0.961561797682962,0.,0.274588618184932));
#13743=DIRECTION('',(-0.961561797682962,0.,-0.274588618184932));
#13744=DIRECTION('',(0.961561797682962,0.,0.274588618184932));
#13745=DIRECTION('',(0.,-1.,0.));
#13746=DIRECTION('center_axis',(0.367515936594704,0.,-0.930017223684012));
#13747=DIRECTION('ref_axis',(0.930017223684012,0.,0.367515936594704));
#13748=DIRECTION('',(-0.930017223684012,0.,-0.367515936594704));
#13749=DIRECTION('',(0.930017223684012,0.,0.367515936594704));
#13750=DIRECTION('',(0.,-1.,0.));
#13751=DIRECTION('center_axis',(0.456903875630421,0.,-0.889516075421856));
#13752=DIRECTION('ref_axis',(0.889516075421856,0.,0.456903875630421));
#13753=DIRECTION('',(-0.889516075421856,0.,-0.456903875630421));
#13754=DIRECTION('',(0.889516075421856,0.,0.456903875630421));
#13755=DIRECTION('',(0.,-1.,0.));
#13756=DIRECTION('center_axis',(0.541891580574752,0.,-0.840448401094438));
#13757=DIRECTION('ref_axis',(0.840448401094438,0.,0.541891580574752));
#13758=DIRECTION('',(-0.840448401094438,0.,-0.541891580574752));
#13759=DIRECTION('',(0.840448401094438,0.,0.541891580574752));
#13760=DIRECTION('',(0.,-1.,0.));
#13761=DIRECTION('center_axis',(0.621660573370078,0.,-0.78328674922865));
#13762=DIRECTION('ref_axis',(0.78328674922865,0.,0.621660573370078));
#13763=DIRECTION('',(-0.78328674922865,0.,-0.621660573370078));
#13764=DIRECTION('',(0.78328674922865,0.,0.621660573370078));
#13765=DIRECTION('',(0.,-1.,0.));
#13766=DIRECTION('center_axis',(0.695442635009612,0.,-0.718581617779697));
#13767=DIRECTION('ref_axis',(0.718581617779697,0.,0.695442635009612));
#13768=DIRECTION('',(-0.718581617779697,0.,-0.695442635009612));
#13769=DIRECTION('',(0.718581617779697,0.,0.695442635009612));
#13770=DIRECTION('',(0.,-1.,0.));
#13771=DIRECTION('center_axis',(0.762527203906389,0.,-0.646956152534857));
#13772=DIRECTION('ref_axis',(0.646956152534857,0.,0.762527203906389));
#13773=DIRECTION('',(-0.646956152534857,0.,-0.762527203906389));
#13774=DIRECTION('',(0.646956152534857,0.,0.762527203906389));
#13775=DIRECTION('',(0.,-1.,0.));
#13776=DIRECTION('center_axis',(-0.60876142900872,0.,-0.793353340291236));
#13777=DIRECTION('ref_axis',(0.793353340291236,0.,-0.60876142900872));
#13778=DIRECTION('',(-0.793353340291236,0.,0.60876142900872));
#13779=DIRECTION('',(0.793353340291236,0.,-0.60876142900872));
#13780=DIRECTION('center_axis',(0.,1.,0.));
#13781=DIRECTION('ref_axis',(-0.5,0.,0.866025403784438));
#13782=DIRECTION('center_axis',(0.,1.,0.));
#13783=DIRECTION('ref_axis',(1.,0.,0.));
#13784=DIRECTION('center_axis',(0.,1.,0.));
#13785=DIRECTION('ref_axis',(1.,0.,0.));
#13786=DIRECTION('center_axis',(0.,1.,0.));
#13787=DIRECTION('ref_axis',(1.,0.,0.));
#13788=DIRECTION('center_axis',(0.,1.,0.));
#13789=DIRECTION('ref_axis',(1.,0.,0.));
#13790=DIRECTION('center_axis',(0.,1.,0.));
#13791=DIRECTION('ref_axis',(1.,0.,0.));
#13792=DIRECTION('center_axis',(0.,1.,0.));
#13793=DIRECTION('ref_axis',(1.,0.,0.));
#13794=DIRECTION('center_axis',(0.,1.,0.));
#13795=DIRECTION('ref_axis',(1.,0.,0.));
#13796=DIRECTION('center_axis',(0.,1.,0.));
#13797=DIRECTION('ref_axis',(1.,0.,0.));
#13798=DIRECTION('center_axis',(0.,1.,0.));
#13799=DIRECTION('ref_axis',(1.,0.,0.));
#13800=DIRECTION('center_axis',(0.,1.,0.));
#13801=DIRECTION('ref_axis',(1.,0.,0.));
#13802=DIRECTION('center_axis',(0.,1.,0.));
#13803=DIRECTION('ref_axis',(1.,0.,0.));
#13804=DIRECTION('center_axis',(0.,1.,0.));
#13805=DIRECTION('ref_axis',(1.,0.,0.));
#13806=DIRECTION('center_axis',(0.,1.,0.));
#13807=DIRECTION('ref_axis',(1.,0.,0.));
#13808=DIRECTION('center_axis',(0.,1.,0.));
#13809=DIRECTION('ref_axis',(1.,0.,0.));
#13810=DIRECTION('center_axis',(0.,1.,0.));
#13811=DIRECTION('ref_axis',(1.,0.,0.));
#13812=DIRECTION('center_axis',(0.,1.,0.));
#13813=DIRECTION('ref_axis',(1.,0.,0.));
#13814=DIRECTION('center_axis',(0.,1.,0.));
#13815=DIRECTION('ref_axis',(1.,0.,0.));
#13816=DIRECTION('center_axis',(0.,1.,0.));
#13817=DIRECTION('ref_axis',(1.,0.,0.));
#13818=DIRECTION('',(-0.923879532511287,0.,-0.38268343236509));
#13819=DIRECTION('',(0.336889853392221,0.,-0.941544065183021));
#13820=DIRECTION('',(0.242980179903264,0.,-0.970031253194544));
#13821=DIRECTION('',(0.146730474455362,0.,-0.989176509964781));
#13822=DIRECTION('',(0.0490676743274181,0.,-0.998795456205172));
#13823=DIRECTION('',(-0.0490676743274181,0.,-0.998795456205172));
#13824=DIRECTION('',(-0.146730474455362,0.,-0.989176509964781));
#13825=DIRECTION('',(-0.242980179903264,0.,-0.970031253194544));
#13826=DIRECTION('',(-0.336889853392221,0.,-0.941544065183021));
#13827=DIRECTION('',(0.923879532511287,0.,-0.38268343236509));
#13828=DIRECTION('center_axis',(0.,1.,0.));
#13829=DIRECTION('ref_axis',(1.,0.,0.));
#13830=DIRECTION('',(0.130526192220051,0.,0.99144486137381));
#13831=DIRECTION('',(-0.983846005927078,0.,0.179016861276632));
#13832=DIRECTION('',(-0.961561797682962,0.,0.274588618184932));
#13833=DIRECTION('',(-0.930017223684012,0.,0.367515936594703));
#13834=DIRECTION('',(-0.889516075421856,0.,0.45690387563042));
#13835=DIRECTION('',(-0.840448401094438,0.,0.541891580574752));
#13836=DIRECTION('',(-0.78328674922865,0.,0.621660573370077));
#13837=DIRECTION('',(-0.718581617779698,0.,0.695442635009612));
#13838=DIRECTION('',(-0.646956152534857,0.,0.762527203906388));
#13839=DIRECTION('',(-0.793353340291235,0.,-0.608761429008721));
#13840=DIRECTION('center_axis',(0.,1.,0.));
#13841=DIRECTION('ref_axis',(1.,0.,0.));
#13842=DIRECTION('center_axis',(0.,1.,0.));
#13843=DIRECTION('ref_axis',(1.,0.,0.));
#13844=DIRECTION('center_axis',(-0.179016861276632,0.,-0.983846005927078));
#13845=DIRECTION('ref_axis',(0.983846005927078,0.,-0.179016861276632));
#13846=DIRECTION('',(-0.983846005927078,0.,0.179016861276632));
#13847=DIRECTION('',(0.,-1.,0.));
#13848=DIRECTION('',(0.983846005927078,0.,-0.179016861276632));
#13849=DIRECTION('',(0.,-1.,0.));
#13850=DIRECTION('center_axis',(-0.274588618184931,0.,-0.961561797682962));
#13851=DIRECTION('ref_axis',(0.961561797682962,0.,-0.274588618184931));
#13852=DIRECTION('',(-0.961561797682962,0.,0.274588618184931));
#13853=DIRECTION('',(0.961561797682962,0.,-0.274588618184931));
#13854=DIRECTION('',(0.,-1.,0.));
#13855=DIRECTION('center_axis',(-0.367515936594702,0.,-0.930017223684013));
#13856=DIRECTION('ref_axis',(0.930017223684013,0.,-0.367515936594702));
#13857=DIRECTION('',(-0.930017223684013,0.,0.367515936594703));
#13858=DIRECTION('',(0.930017223684013,0.,-0.367515936594702));
#13859=DIRECTION('',(0.,-1.,0.));
#13860=DIRECTION('center_axis',(-0.456903875630422,0.,-0.889516075421855));
#13861=DIRECTION('ref_axis',(0.889516075421855,0.,-0.456903875630422));
#13862=DIRECTION('',(-0.889516075421855,0.,0.456903875630422));
#13863=DIRECTION('',(0.889516075421855,0.,-0.456903875630422));
#13864=DIRECTION('',(0.,-1.,0.));
#13865=DIRECTION('center_axis',(-0.54189158057475,0.,-0.840448401094439));
#13866=DIRECTION('ref_axis',(0.840448401094439,0.,-0.54189158057475));
#13867=DIRECTION('',(-0.840448401094439,0.,0.54189158057475));
#13868=DIRECTION('',(0.840448401094439,0.,-0.54189158057475));
#13869=DIRECTION('',(0.,-1.,0.));
#13870=DIRECTION('center_axis',(-0.621660573370078,0.,-0.78328674922865));
#13871=DIRECTION('ref_axis',(0.78328674922865,0.,-0.621660573370078));
#13872=DIRECTION('',(-0.78328674922865,0.,0.621660573370078));
#13873=DIRECTION('',(0.78328674922865,0.,-0.621660573370078));
#13874=DIRECTION('',(0.,-1.,0.));
#13875=DIRECTION('center_axis',(-0.695442635009612,0.,-0.718581617779698));
#13876=DIRECTION('ref_axis',(0.718581617779698,0.,-0.695442635009612));
#13877=DIRECTION('',(-0.718581617779698,0.,0.695442635009612));
#13878=DIRECTION('',(0.718581617779698,0.,-0.695442635009612));
#13879=DIRECTION('',(0.,-1.,0.));
#13880=DIRECTION('center_axis',(-0.762527203906389,0.,-0.646956152534857));
#13881=DIRECTION('ref_axis',(0.646956152534857,0.,-0.762527203906389));
#13882=DIRECTION('',(-0.646956152534857,0.,0.762527203906389));
#13883=DIRECTION('',(0.646956152534857,0.,-0.762527203906389));
#13884=DIRECTION('',(0.,-1.,0.));
#13885=DIRECTION('center_axis',(-0.608761429008721,0.,0.793353340291235));
#13886=DIRECTION('ref_axis',(-0.793353340291235,0.,-0.608761429008721));
#13887=DIRECTION('',(0.793353340291235,0.,0.608761429008721));
#13888=DIRECTION('',(0.,-1.,0.));
#13889=DIRECTION('center_axis',(0.762527203906388,0.,0.646956152534857));
#13890=DIRECTION('ref_axis',(-0.646956152534857,0.,0.762527203906388));
#13891=DIRECTION('',(0.646956152534857,0.,-0.762527203906388));
#13892=DIRECTION('',(0.,-1.,0.));
#13893=DIRECTION('center_axis',(0.695442635009612,0.,0.718581617779698));
#13894=DIRECTION('ref_axis',(-0.718581617779698,0.,0.695442635009612));
#13895=DIRECTION('',(0.718581617779698,0.,-0.695442635009612));
#13896=DIRECTION('',(0.,-1.,0.));
#13897=DIRECTION('center_axis',(0.621660573370077,0.,0.78328674922865));
#13898=DIRECTION('ref_axis',(-0.78328674922865,0.,0.621660573370077));
#13899=DIRECTION('',(0.78328674922865,0.,-0.621660573370077));
#13900=DIRECTION('',(0.,-1.,0.));
#13901=DIRECTION('center_axis',(0.541891580574752,0.,0.840448401094438));
#13902=DIRECTION('ref_axis',(-0.840448401094438,0.,0.541891580574752));
#13903=DIRECTION('',(0.840448401094438,0.,-0.541891580574752));
#13904=DIRECTION('',(0.,-1.,0.));
#13905=DIRECTION('center_axis',(0.45690387563042,0.,0.889516075421856));
#13906=DIRECTION('ref_axis',(-0.889516075421856,0.,0.45690387563042));
#13907=DIRECTION('',(0.889516075421856,0.,-0.45690387563042));
#13908=DIRECTION('',(0.,-1.,0.));
#13909=DIRECTION('center_axis',(0.367515936594703,0.,0.930017223684012));
#13910=DIRECTION('ref_axis',(-0.930017223684012,0.,0.367515936594703));
#13911=DIRECTION('',(0.930017223684012,0.,-0.367515936594703));
#13912=DIRECTION('',(0.,-1.,0.));
#13913=DIRECTION('center_axis',(0.274588618184932,0.,0.961561797682962));
#13914=DIRECTION('ref_axis',(-0.961561797682962,0.,0.274588618184932));
#13915=DIRECTION('',(0.961561797682962,0.,-0.274588618184932));
#13916=DIRECTION('',(0.,-1.,0.));
#13917=DIRECTION('center_axis',(0.179016861276632,0.,0.983846005927078));
#13918=DIRECTION('ref_axis',(-0.983846005927078,0.,0.179016861276632));
#13919=DIRECTION('',(0.983846005927078,0.,-0.179016861276632));
#13920=DIRECTION('',(0.,-1.,0.));
#13921=DIRECTION('center_axis',(0.99144486137381,0.,-0.130526192220051));
#13922=DIRECTION('ref_axis',(0.130526192220051,0.,0.99144486137381));
#13923=DIRECTION('',(-0.130526192220051,0.,-0.99144486137381));
#13924=DIRECTION('center_axis',(0.,1.,0.));
#13925=DIRECTION('ref_axis',(-0.5,0.,-0.866025403784439));
#13926=DIRECTION('center_axis',(0.,1.,0.));
#13927=DIRECTION('ref_axis',(1.,0.,0.));
#13928=DIRECTION('center_axis',(0.,1.,0.));
#13929=DIRECTION('ref_axis',(1.,0.,0.));
#13930=DIRECTION('center_axis',(0.,1.,0.));
#13931=DIRECTION('ref_axis',(1.,0.,0.));
#13932=DIRECTION('center_axis',(0.,1.,0.));
#13933=DIRECTION('ref_axis',(1.,0.,0.));
#13934=DIRECTION('center_axis',(0.,1.,0.));
#13935=DIRECTION('ref_axis',(1.,0.,0.));
#13936=DIRECTION('center_axis',(0.,1.,0.));
#13937=DIRECTION('ref_axis',(1.,0.,0.));
#13938=DIRECTION('center_axis',(0.,1.,0.));
#13939=DIRECTION('ref_axis',(1.,0.,0.));
#13940=DIRECTION('center_axis',(0.,1.,0.));
#13941=DIRECTION('ref_axis',(1.,0.,0.));
#13942=DIRECTION('center_axis',(0.,1.,0.));
#13943=DIRECTION('ref_axis',(1.,0.,0.));
#13944=DIRECTION('center_axis',(0.,1.,0.));
#13945=DIRECTION('ref_axis',(1.,0.,0.));
#13946=DIRECTION('center_axis',(0.,1.,0.));
#13947=DIRECTION('ref_axis',(1.,0.,0.));
#13948=DIRECTION('center_axis',(0.,1.,0.));
#13949=DIRECTION('ref_axis',(1.,0.,0.));
#13950=DIRECTION('center_axis',(0.,1.,0.));
#13951=DIRECTION('ref_axis',(1.,0.,0.));
#13952=DIRECTION('center_axis',(0.,1.,0.));
#13953=DIRECTION('ref_axis',(1.,0.,0.));
#13954=DIRECTION('center_axis',(0.,1.,0.));
#13955=DIRECTION('ref_axis',(1.,0.,0.));
#13956=DIRECTION('center_axis',(0.,1.,0.));
#13957=DIRECTION('ref_axis',(1.,0.,0.));
#13958=DIRECTION('center_axis',(0.94154406518302,0.,0.336889853392221));
#13959=DIRECTION('ref_axis',(-0.336889853392221,0.,0.94154406518302));
#13960=DIRECTION('',(0.336889853392221,0.,-0.94154406518302));
#13961=DIRECTION('',(0.,-1.,0.));
#13962=DIRECTION('',(-0.336889853392221,0.,0.94154406518302));
#13963=DIRECTION('',(0.,-1.,0.));
#13964=DIRECTION('center_axis',(0.970031253194544,0.,0.242980179903265));
#13965=DIRECTION('ref_axis',(-0.242980179903265,0.,0.970031253194544));
#13966=DIRECTION('',(0.242980179903265,0.,-0.970031253194544));
#13967=DIRECTION('',(-0.242980179903265,0.,0.970031253194544));
#13968=DIRECTION('',(0.,-1.,0.));
#13969=DIRECTION('center_axis',(0.989176509964781,0.,0.146730474455363));
#13970=DIRECTION('ref_axis',(-0.146730474455363,0.,0.989176509964781));
#13971=DIRECTION('',(0.146730474455363,0.,-0.989176509964781));
#13972=DIRECTION('',(-0.146730474455363,0.,0.989176509964781));
#13973=DIRECTION('',(0.,-1.,0.));
#13974=DIRECTION('center_axis',(0.998795456205173,0.,0.049067674327416));
#13975=DIRECTION('ref_axis',(-0.049067674327416,0.,0.998795456205173));
#13976=DIRECTION('',(0.049067674327416,0.,-0.998795456205173));
#13977=DIRECTION('',(-0.049067674327416,0.,0.998795456205173));
#13978=DIRECTION('',(0.,-1.,0.));
#13979=DIRECTION('center_axis',(0.998795456205173,0.,-0.049067674327416));
#13980=DIRECTION('ref_axis',(0.049067674327416,0.,0.998795456205173));
#13981=DIRECTION('',(-0.049067674327416,0.,-0.998795456205173));
#13982=DIRECTION('',(0.049067674327416,0.,0.998795456205173));
#13983=DIRECTION('',(0.,-1.,0.));
#13984=DIRECTION('center_axis',(0.989176509964781,0.,-0.146730474455363));
#13985=DIRECTION('ref_axis',(0.146730474455363,0.,0.989176509964781));
#13986=DIRECTION('',(-0.146730474455363,0.,-0.989176509964781));
#13987=DIRECTION('',(0.146730474455363,0.,0.989176509964781));
#13988=DIRECTION('',(0.,-1.,0.));
#13989=DIRECTION('center_axis',(0.970031253194544,0.,-0.242980179903265));
#13990=DIRECTION('ref_axis',(0.242980179903265,0.,0.970031253194544));
#13991=DIRECTION('',(-0.242980179903265,0.,-0.970031253194544));
#13992=DIRECTION('',(0.242980179903265,0.,0.970031253194544));
#13993=DIRECTION('',(0.,-1.,0.));
#13994=DIRECTION('center_axis',(0.94154406518302,0.,-0.336889853392221));
#13995=DIRECTION('ref_axis',(0.336889853392221,0.,0.94154406518302));
#13996=DIRECTION('',(-0.336889853392221,0.,-0.94154406518302));
#13997=DIRECTION('',(0.336889853392221,0.,0.94154406518302));
#13998=DIRECTION('',(0.,-1.,0.));
#13999=DIRECTION('center_axis',(-0.38268343236509,0.,-0.923879532511287));
#14000=DIRECTION('ref_axis',(0.923879532511287,0.,-0.38268343236509));
#14001=DIRECTION('',(-0.923879532511287,0.,0.38268343236509));
#14002=DIRECTION('',(0.,-1.,0.));
#14003=DIRECTION('center_axis',(-0.941544065183021,0.,0.336889853392221));
#14004=DIRECTION('ref_axis',(-0.336889853392221,0.,-0.941544065183021));
#14005=DIRECTION('',(0.336889853392221,0.,0.941544065183021));
#14006=DIRECTION('',(0.,-1.,0.));
#14007=DIRECTION('center_axis',(-0.970031253194544,0.,0.242980179903264));
#14008=DIRECTION('ref_axis',(-0.242980179903264,0.,-0.970031253194544));
#14009=DIRECTION('',(0.242980179903264,0.,0.970031253194544));
#14010=DIRECTION('',(0.,-1.,0.));
#14011=DIRECTION('center_axis',(-0.989176509964781,0.,0.146730474455362));
#14012=DIRECTION('ref_axis',(-0.146730474455362,0.,-0.989176509964781));
#14013=DIRECTION('',(0.146730474455362,0.,0.989176509964781));
#14014=DIRECTION('',(0.,-1.,0.));
#14015=DIRECTION('center_axis',(-0.998795456205172,0.,0.0490676743274181));
#14016=DIRECTION('ref_axis',(-0.0490676743274181,0.,-0.998795456205172));
#14017=DIRECTION('',(0.0490676743274181,0.,0.998795456205172));
#14018=DIRECTION('',(0.,-1.,0.));
#14019=DIRECTION('center_axis',(-0.998795456205172,0.,-0.0490676743274181));
#14020=DIRECTION('ref_axis',(0.0490676743274181,0.,-0.998795456205172));
#14021=DIRECTION('',(-0.0490676743274181,0.,0.998795456205172));
#14022=DIRECTION('',(0.,-1.,0.));
#14023=DIRECTION('center_axis',(-0.989176509964781,0.,-0.146730474455362));
#14024=DIRECTION('ref_axis',(0.146730474455362,0.,-0.989176509964781));
#14025=DIRECTION('',(-0.146730474455362,0.,0.989176509964781));
#14026=DIRECTION('',(0.,-1.,0.));
#14027=DIRECTION('center_axis',(-0.970031253194544,0.,-0.242980179903264));
#14028=DIRECTION('ref_axis',(0.242980179903264,0.,-0.970031253194544));
#14029=DIRECTION('',(-0.242980179903264,0.,0.970031253194544));
#14030=DIRECTION('',(0.,-1.,0.));
#14031=DIRECTION('center_axis',(-0.941544065183021,0.,-0.336889853392221));
#14032=DIRECTION('ref_axis',(0.336889853392221,0.,-0.941544065183021));
#14033=DIRECTION('',(-0.336889853392221,0.,0.941544065183021));
#14034=DIRECTION('',(0.,-1.,0.));
#14035=DIRECTION('center_axis',(-0.38268343236509,0.,0.923879532511287));
#14036=DIRECTION('ref_axis',(-0.923879532511287,0.,-0.38268343236509));
#14037=DIRECTION('',(0.923879532511287,0.,0.38268343236509));
#14038=DIRECTION('center_axis',(0.,1.,0.));
#14039=DIRECTION('ref_axis',(1.,0.,0.));
#14040=DIRECTION('center_axis',(0.,1.,0.));
#14041=DIRECTION('ref_axis',(1.,0.,0.));
#14042=DIRECTION('center_axis',(0.,1.,0.));
#14043=DIRECTION('ref_axis',(1.,0.,0.));
#14044=DIRECTION('center_axis',(0.,1.,0.));
#14045=DIRECTION('ref_axis',(1.,0.,0.));
#14046=DIRECTION('center_axis',(0.,1.,0.));
#14047=DIRECTION('ref_axis',(1.,0.,0.));
#14048=DIRECTION('center_axis',(0.,1.,0.));
#14049=DIRECTION('ref_axis',(1.,0.,0.));
#14050=DIRECTION('center_axis',(0.,1.,0.));
#14051=DIRECTION('ref_axis',(1.,0.,0.));
#14052=DIRECTION('center_axis',(0.,1.,0.));
#14053=DIRECTION('ref_axis',(1.,0.,0.));
#14054=DIRECTION('center_axis',(0.,1.,0.));
#14055=DIRECTION('ref_axis',(1.,0.,0.));
#14056=DIRECTION('center_axis',(0.,1.,0.));
#14057=DIRECTION('ref_axis',(1.,0.,0.));
#14058=DIRECTION('center_axis',(0.,1.,0.));
#14059=DIRECTION('ref_axis',(1.,0.,0.));
#14060=DIRECTION('center_axis',(0.,1.,0.));
#14061=DIRECTION('ref_axis',(1.,0.,0.));
#14062=DIRECTION('center_axis',(0.,1.,0.));
#14063=DIRECTION('ref_axis',(1.,0.,0.));
#14064=DIRECTION('center_axis',(0.,1.,0.));
#14065=DIRECTION('ref_axis',(1.,0.,0.));
#14066=DIRECTION('center_axis',(0.,1.,0.));
#14067=DIRECTION('ref_axis',(1.,0.,0.));
#14068=DIRECTION('center_axis',(0.,1.,0.));
#14069=DIRECTION('ref_axis',(1.,0.,0.));
#14070=DIRECTION('center_axis',(0.,1.,0.));
#14071=DIRECTION('ref_axis',(1.,0.,0.));
#14072=DIRECTION('center_axis',(0.,-1.,0.));
#14073=DIRECTION('ref_axis',(1.,0.,0.));
#14074=DIRECTION('center_axis',(0.,-1.,0.));
#14075=DIRECTION('ref_axis',(1.,0.,0.));
#14076=DIRECTION('',(0.,1.,0.));
#14077=DIRECTION('center_axis',(0.,1.,0.));
#14078=DIRECTION('ref_axis',(1.,0.,0.));
#17312=CARTESIAN_POINT('',(0.,0.,0.));
#17313=CARTESIAN_POINT('Origin',(0.,-1.525,0.));
#17314=CARTESIAN_POINT('',(0.21,-1.525,0.562049819855856));
#17315=CARTESIAN_POINT('',(-0.21,-1.525,0.562049819855856));
#17316=CARTESIAN_POINT('Ctrl Pts',(0.21,-1.525,0.562049819855856));
#17317=CARTESIAN_POINT('Ctrl Pts',(0.21,-1.49837871751922,0.562049819855856));
#17318=CARTESIAN_POINT('Ctrl Pts',(0.204633348688358,-1.4701551027118,0.564140225270058));
#17319=CARTESIAN_POINT('Ctrl Pts',(0.183136586201564,-1.41849286725608,
0.571480520223595));
#17320=CARTESIAN_POINT('Ctrl Pts',(0.167016776838808,-1.39503192874046,
0.576602928616412));
#17321=CARTESIAN_POINT('Ctrl Pts',(0.129978636309075,-1.35799378821073,
0.586063715219224));
#17322=CARTESIAN_POINT('Ctrl Pts',(0.106513536936886,-1.34186587223919,
0.591045521796147));
#17323=CARTESIAN_POINT('Ctrl Pts',(0.0548356965671431,-1.32036302924048,
0.598057680137));
#17324=CARTESIAN_POINT('Ctrl Pts',(0.0266060994851219,-1.315,0.6));
#17325=CARTESIAN_POINT('Ctrl Pts',(-0.026606099485122,-1.315,0.6));
#17326=CARTESIAN_POINT('Ctrl Pts',(-0.0548356965671431,-1.32036302924048,
0.598057680137));
#17327=CARTESIAN_POINT('Ctrl Pts',(-0.106513536936886,-1.34186587223919,
0.591045521796147));
#17328=CARTESIAN_POINT('Ctrl Pts',(-0.129978636309075,-1.35799378821073,
0.586063715219224));
#17329=CARTESIAN_POINT('Ctrl Pts',(-0.167016776838808,-1.39503192874046,
0.576602928616412));
#17330=CARTESIAN_POINT('Ctrl Pts',(-0.183136586201564,-1.41849286725608,
0.571480520223595));
#17331=CARTESIAN_POINT('Ctrl Pts',(-0.204633348688358,-1.4701551027118,
0.564140225270058));
#17332=CARTESIAN_POINT('Ctrl Pts',(-0.21,-1.49837871751922,0.562049819855856));
#17333=CARTESIAN_POINT('Ctrl Pts',(-0.21,-1.525,0.562049819855856));
#17334=CARTESIAN_POINT('Ctrl Pts',(-0.21,-1.525,0.562049819855856));
#17335=CARTESIAN_POINT('Ctrl Pts',(-0.21,-1.55162128248078,0.562049819855856));
#17336=CARTESIAN_POINT('Ctrl Pts',(-0.204633348688358,-1.5798448972882,
0.564140225270058));
#17337=CARTESIAN_POINT('Ctrl Pts',(-0.183136586201564,-1.63150713274392,
0.571480520223595));
#17338=CARTESIAN_POINT('Ctrl Pts',(-0.167016776838808,-1.65496807125954,
0.576602928616412));
#17339=CARTESIAN_POINT('Ctrl Pts',(-0.129978636309075,-1.69200621178927,
0.586063715219224));
#17340=CARTESIAN_POINT('Ctrl Pts',(-0.106513536936886,-1.70813412776081,
0.591045521796147));
#17341=CARTESIAN_POINT('Ctrl Pts',(-0.0548356965671429,-1.72963697075952,
0.598057680137));
#17342=CARTESIAN_POINT('Ctrl Pts',(-0.026606099485122,-1.735,0.6));
#17343=CARTESIAN_POINT('Ctrl Pts',(0.026606099485122,-1.735,0.6));
#17344=CARTESIAN_POINT('Ctrl Pts',(0.0548356965671429,-1.72963697075952,
0.598057680137));
#17345=CARTESIAN_POINT('Ctrl Pts',(0.106513536936886,-1.70813412776081,
0.591045521796147));
#17346=CARTESIAN_POINT('Ctrl Pts',(0.129978636309075,-1.69200621178927,
0.586063715219224));
#17347=CARTESIAN_POINT('Ctrl Pts',(0.167016776838808,-1.65496807125954,
0.576602928616412));
#17348=CARTESIAN_POINT('Ctrl Pts',(0.183136586201564,-1.63150713274392,
0.571480520223595));
#17349=CARTESIAN_POINT('Ctrl Pts',(0.204633348688358,-1.5798448972882,0.564140225270058));
#17350=CARTESIAN_POINT('Ctrl Pts',(0.21,-1.55162128248078,0.562049819855856));
#17351=CARTESIAN_POINT('Ctrl Pts',(0.21,-1.525,0.562049819855856));
#17352=CARTESIAN_POINT('',(-0.21,-1.525,1.35380944006164));
#17353=CARTESIAN_POINT('',(-0.21,-1.525,0.));
#17354=CARTESIAN_POINT('Ctrl Pts',(-0.21,-1.525,1.35380944006164));
#17355=CARTESIAN_POINT('Ctrl Pts',(-0.21,-1.49858689919462,1.35380944006164));
#17356=CARTESIAN_POINT('Ctrl Pts',(-0.204712795751841,-1.47044219200607,
1.35466231450937));
#17357=CARTESIAN_POINT('Ctrl Pts',(-0.183268700413686,-1.41871515620915,
1.35772968493193));
#17358=CARTESIAN_POINT('Ctrl Pts',(-0.167114046419118,-1.39512919832077,
1.35989844568037));
#17359=CARTESIAN_POINT('Ctrl Pts',(-0.129871156089225,-1.35788630799087,
1.36395907436197));
#17360=CARTESIAN_POINT('Ctrl Pts',(-0.106285045427176,-1.34173137598416,
1.36611666311719));
#17361=CARTESIAN_POINT('Ctrl Pts',(-0.0545574871667227,-1.32028707843824,
1.36915840160825));
#17362=CARTESIAN_POINT('Ctrl Pts',(-0.026412598106597,-1.315,1.37));
#17363=CARTESIAN_POINT('Ctrl Pts',(0.0264125981065971,-1.315,1.37));
#17364=CARTESIAN_POINT('Ctrl Pts',(0.0545574871667228,-1.32028707843824,
1.36915840160825));
#17365=CARTESIAN_POINT('Ctrl Pts',(0.106285045427176,-1.34173137598416,
1.36611666311719));
#17366=CARTESIAN_POINT('Ctrl Pts',(0.129871156089225,-1.35788630799087,
1.36395907436197));
#17367=CARTESIAN_POINT('Ctrl Pts',(0.167114046419118,-1.39512919832077,
1.35989844568037));
#17368=CARTESIAN_POINT('Ctrl Pts',(0.183268700413687,-1.41871515620915,
1.35772968493193));
#17369=CARTESIAN_POINT('Ctrl Pts',(0.204712795751841,-1.47044219200607,
1.35466231450937));
#17370=CARTESIAN_POINT('Ctrl Pts',(0.21,-1.49858689919462,1.35380944006164));
#17371=CARTESIAN_POINT('Ctrl Pts',(0.21,-1.55141310080538,1.35380944006164));
#17372=CARTESIAN_POINT('Ctrl Pts',(0.204712795751841,-1.57955780799393,
1.35466231450937));
#17373=CARTESIAN_POINT('Ctrl Pts',(0.183268700413686,-1.63128484379085,
1.35772968493193));
#17374=CARTESIAN_POINT('Ctrl Pts',(0.167114046419118,-1.65487080167923,
1.35989844568037));
#17375=CARTESIAN_POINT('Ctrl Pts',(0.129871156089225,-1.69211369200913,
1.36395907436197));
#17376=CARTESIAN_POINT('Ctrl Pts',(0.106285045427176,-1.70826862401584,
1.36611666311719));
#17377=CARTESIAN_POINT('Ctrl Pts',(0.0545574871667227,-1.72971292156176,
1.36915840160825));
#17378=CARTESIAN_POINT('Ctrl Pts',(0.0264125981065971,-1.735,1.37));
#17379=CARTESIAN_POINT('Ctrl Pts',(-0.026412598106597,-1.735,1.37));
#17380=CARTESIAN_POINT('Ctrl Pts',(-0.0545574871667227,-1.72971292156176,
1.36915840160825));
#17381=CARTESIAN_POINT('Ctrl Pts',(-0.106285045427176,-1.70826862401584,
1.36611666311719));
#17382=CARTESIAN_POINT('Ctrl Pts',(-0.129871156089225,-1.69211369200912,
1.36395907436197));
#17383=CARTESIAN_POINT('Ctrl Pts',(-0.167114046419118,-1.65487080167923,
1.35989844568037));
#17384=CARTESIAN_POINT('Ctrl Pts',(-0.183268700413686,-1.63128484379085,
1.35772968493193));
#17385=CARTESIAN_POINT('Ctrl Pts',(-0.204712795751841,-1.57955780799393,
1.35466231450937));
#17386=CARTESIAN_POINT('Ctrl Pts',(-0.21,-1.55141310080538,1.35380944006164));
#17387=CARTESIAN_POINT('Ctrl Pts',(-0.21,-1.525,1.35380944006164));
#17388=CARTESIAN_POINT('Origin',(0.,0.,0.));
#17389=CARTESIAN_POINT('',(-0.6,-2.05,7.34788079488412E-17));
#17390=CARTESIAN_POINT('Origin',(0.,-2.05,0.));
#17391=CARTESIAN_POINT('',(-0.6,-1.,-7.34788079488412E-17));
#17392=CARTESIAN_POINT('',(-0.6,0.,7.34788079488412E-17));
#17393=CARTESIAN_POINT('Origin',(0.,-1.,0.));
#17394=CARTESIAN_POINT('Origin',(-0.999913779596035,-0.4,0.936521453771333));
#17395=CARTESIAN_POINT('',(-1.08689407619899,-0.4,0.834003157741947));
#17396=CARTESIAN_POINT('',(-0.999913779596035,-0.4,0.936521453771333));
#17397=CARTESIAN_POINT('',(-1.08689407619899,-0.4,0.834003157741947));
#17398=CARTESIAN_POINT('',(-1.08689407619899,-1.,0.834003157741947));
#17399=CARTESIAN_POINT('',(-1.08689407619899,-0.4,0.834003157741947));
#17400=CARTESIAN_POINT('',(-0.999913779596035,-1.,0.936521453771333));
#17401=CARTESIAN_POINT('',(-1.02165885374678,-1.,0.910891879763986));
#17402=CARTESIAN_POINT('',(-0.999913779596035,-0.4,0.936521453771333));
#17403=CARTESIAN_POINT('Origin',(-0.903303766687095,-0.4,1.0300205362462));
#17404=CARTESIAN_POINT('',(-0.903303766687095,-0.4,1.0300205362462));
#17405=CARTESIAN_POINT('',(-0.999913779596035,-0.4,0.936521453771333));
#17406=CARTESIAN_POINT('',(-0.903303766687095,-1.,1.0300205362462));
#17407=CARTESIAN_POINT('',(-0.92745626991433,-1.,1.00664576562748));
#17408=CARTESIAN_POINT('',(-0.903303766687095,-0.4,1.0300205362462));
#17409=CARTESIAN_POINT('Origin',(-0.79799444470889,-0.4,1.11359995789051));
#17410=CARTESIAN_POINT('',(-0.79799444470889,-0.4,1.11359995789051));
#17411=CARTESIAN_POINT('',(-0.903303766687095,-0.4,1.0300205362462));
#17412=CARTESIAN_POINT('',(-0.79799444470889,-1.,1.11359995789051));
#17413=CARTESIAN_POINT('',(-0.824321775203442,-1.,1.09270510247943));
#17414=CARTESIAN_POINT('',(-0.79799444470889,-0.4,1.11359995789051));
#17415=CARTESIAN_POINT('Origin',(-0.685,-0.4,1.18645480318468));
#17416=CARTESIAN_POINT('',(-0.685,-0.4,1.18645480318468));
#17417=CARTESIAN_POINT('',(-0.79799444470889,-0.4,1.11359995789051));
#17418=CARTESIAN_POINT('',(-0.685,-1.,1.18645480318468));
#17419=CARTESIAN_POINT('',(-0.713248611177222,-1.,1.16824109186114));
#17420=CARTESIAN_POINT('',(-0.685,-0.4,1.18645480318468));
#17421=CARTESIAN_POINT('Origin',(-0.565408630832021,-0.4,1.24788344014201));
#17422=CARTESIAN_POINT('',(-0.565408630832021,-0.4,1.24788344014201));
#17423=CARTESIAN_POINT('',(-0.685,-0.4,1.18645480318468));
#17424=CARTESIAN_POINT('',(-0.565408630832022,-1.,1.24788344014201));
#17425=CARTESIAN_POINT('',(-0.595306473124018,-1.,1.23252628090268));
#17426=CARTESIAN_POINT('',(-0.565408630832021,-0.4,1.24788344014201));
#17427=CARTESIAN_POINT('Origin',(-0.440372067465332,-0.4,1.29729427740829));
#17428=CARTESIAN_POINT('',(-0.440372067465332,-0.4,1.29729427740829));
#17429=CARTESIAN_POINT('',(-0.565408630832021,-0.4,1.24788344014201));
#17430=CARTESIAN_POINT('',(-0.440372067465332,-1.,1.29729427740829));
#17431=CARTESIAN_POINT('',(-0.471631208307004,-1.,1.28494156809172));
#17432=CARTESIAN_POINT('',(-0.440372067465332,-0.4,1.29729427740829));
#17433=CARTESIAN_POINT('Origin',(-0.311094480357092,-0.4,1.33421146160995));
#17434=CARTESIAN_POINT('',(-0.311094480357092,-0.4,1.33421146160995));
#17435=CARTESIAN_POINT('',(-0.440372067465332,-0.4,1.29729427740829));
#17436=CARTESIAN_POINT('',(-0.311094480357092,-1.,1.33421146160995));
#17437=CARTESIAN_POINT('',(-0.343413877134152,-1.,1.32498216555953));
#17438=CARTESIAN_POINT('',(-0.311094480357092,-0.4,1.33421146160995));
#17439=CARTESIAN_POINT('Origin',(-0.178820883341471,-0.4,1.35827946008212));
#17440=CARTESIAN_POINT('',(-0.178820883341471,-0.4,1.35827946008212));
#17441=CARTESIAN_POINT('',(-0.311094480357092,-0.4,1.33421146160995));
#17442=CARTESIAN_POINT('',(-0.178820883341471,-1.,1.35827946008212));
#17443=CARTESIAN_POINT('',(-0.211889282595376,-1.,1.35226246046408));
#17444=CARTESIAN_POINT('',(-0.178820883341471,-0.4,1.35827946008212));
#17445=CARTESIAN_POINT('Origin',(-0.104420953776042,-0.4,0.793155889099048));
#17446=CARTESIAN_POINT('',(-0.104420953776042,-0.4,0.793155889099048));
#17447=CARTESIAN_POINT('',(-0.178820883341471,-0.4,1.35827946008212));
#17448=CARTESIAN_POINT('',(-0.104420953776042,-1.,0.793155889099048));
#17449=CARTESIAN_POINT('',(-0.0522104768880209,-1.,0.396577944549524));
#17450=CARTESIAN_POINT('',(-0.104420953776042,-0.4,0.793155889099048));
#17451=CARTESIAN_POINT('Origin',(-0.181661010427499,-0.4,0.779101583421867));
#17452=CARTESIAN_POINT('',(-0.181661010427499,-0.4,0.779101583421867));
#17453=CARTESIAN_POINT('',(-0.104420953776042,-0.4,0.793155889099048));
#17454=CARTESIAN_POINT('',(-0.181661010427499,-1.,0.779101583421867));
#17455=CARTESIAN_POINT('',(-0.162350996264634,-1.,0.782615159841162));
#17456=CARTESIAN_POINT('',(-0.181661010427499,-0.4,0.779101583421867));
#17457=CARTESIAN_POINT('Origin',(-0.25715157224253,-0.4,0.757544103596084));
#17458=CARTESIAN_POINT('',(-0.25715157224253,-0.4,0.757544103596084));
#17459=CARTESIAN_POINT('',(-0.181661010427499,-0.4,0.779101583421867));
#17460=CARTESIAN_POINT('',(-0.25715157224253,-1.,0.757544103596084));
#17461=CARTESIAN_POINT('',(-0.238278931788772,-1.,0.76293347355253));
#17462=CARTESIAN_POINT('',(-0.25715157224253,-0.4,0.757544103596084));
#17463=CARTESIAN_POINT('Origin',(-0.330165623843516,-0.4,0.72869105993694));
#17464=CARTESIAN_POINT('',(-0.330165623843516,-0.4,0.72869105993694));
#17465=CARTESIAN_POINT('',(-0.25715157224253,-0.4,0.757544103596084));
#17466=CARTESIAN_POINT('',(-0.330165623843516,-1.,0.72869105993694));
#17467=CARTESIAN_POINT('',(-0.311912110943269,-1.,0.735904320851726));
#17468=CARTESIAN_POINT('',(-0.330165623843516,-0.4,0.72869105993694));
#17469=CARTESIAN_POINT('Origin',(-0.4,-0.4,0.692820323027551));
#17470=CARTESIAN_POINT('',(-0.4,-0.4,0.692820323027551));
#17471=CARTESIAN_POINT('',(-0.330165623843516,-0.4,0.72869105993694));
#17472=CARTESIAN_POINT('',(-0.4,-1.,0.692820323027551));
#17473=CARTESIAN_POINT('',(-0.382541405960879,-1.,0.701788007254898));
#17474=CARTESIAN_POINT('',(-0.4,-0.4,0.692820323027551));
#17475=CARTESIAN_POINT('Origin',(-0.465982157494242,-0.4,0.650277347673292));
#17476=CARTESIAN_POINT('',(-0.465982157494242,-0.4,0.650277347673292));
#17477=CARTESIAN_POINT('',(-0.4,-0.4,0.692820323027551));
#17478=CARTESIAN_POINT('',(-0.465982157494242,-1.,0.650277347673292));
#17479=CARTESIAN_POINT('',(-0.449486618120682,-1.,0.660913091511857));
#17480=CARTESIAN_POINT('',(-0.465982157494242,-0.4,0.650277347673292));
#17481=CARTESIAN_POINT('Origin',(-0.527476652080055,-0.4,0.601471845983182));
#17482=CARTESIAN_POINT('',(-0.527476652080055,-0.4,0.601471845983182));
#17483=CARTESIAN_POINT('',(-0.465982157494242,-0.4,0.650277347673292));
#17484=CARTESIAN_POINT('',(-0.527476652080055,-1.,0.601471845983182));
#17485=CARTESIAN_POINT('',(-0.512103028433602,-1.,0.613673221405709));
#17486=CARTESIAN_POINT('',(-0.527476652080055,-0.4,0.601471845983182));
#17487=CARTESIAN_POINT('Origin',(-0.583891258158269,-0.4,0.546873841618297));
#17488=CARTESIAN_POINT('',(-0.583891258158269,-0.4,0.546873841618297));
#17489=CARTESIAN_POINT('',(-0.527476652080055,-0.4,0.601471845983182));
#17490=CARTESIAN_POINT('',(-0.583891258158269,-1.,0.546873841618297));
#17491=CARTESIAN_POINT('',(-0.569787606638716,-1.,0.560523342709518));
#17492=CARTESIAN_POINT('',(-0.583891258158269,-0.4,0.546873841618297));
#17493=CARTESIAN_POINT('Origin',(-0.634682672232988,-0.4,0.487009143206976));
#17494=CARTESIAN_POINT('',(-0.634682672232988,-0.4,0.487009143206976));
#17495=CARTESIAN_POINT('',(-0.583891258158269,-0.4,0.546873841618297));
#17496=CARTESIAN_POINT('',(-0.634682672232988,-1.,0.487009143206976));
#17497=CARTESIAN_POINT('',(-0.621984818714309,-1.,0.501975317809806));
#17498=CARTESIAN_POINT('',(-0.634682672232988,-0.4,0.487009143206976));
#17499=CARTESIAN_POINT('Origin',(-1.08689407619899,-0.4,0.834003157741947));
#17500=CARTESIAN_POINT('',(-0.634682672232988,-0.4,0.487009143206976));
#17501=CARTESIAN_POINT('',(-0.543447038099496,-1.,0.417001578870973));
#17502=CARTESIAN_POINT('Origin',(-0.527275906502258,-0.4,0.913268659668846));
#17503=CARTESIAN_POINT('Origin',(0.,-1.,0.));
#17504=CARTESIAN_POINT('Origin',(0.,-1.,0.));
#17505=CARTESIAN_POINT('Origin',(0.,-1.,0.));
#17506=CARTESIAN_POINT('Origin',(0.,-1.,0.));
#17507=CARTESIAN_POINT('Origin',(0.,-1.,0.));
#17508=CARTESIAN_POINT('Origin',(0.,-1.,0.));
#17509=CARTESIAN_POINT('Origin',(0.,-1.,0.));
#17510=CARTESIAN_POINT('Origin',(0.,-1.,0.));
#17511=CARTESIAN_POINT('Origin',(0.,-1.,0.));
#17512=CARTESIAN_POINT('Origin',(0.,-1.,0.));
#17513=CARTESIAN_POINT('Origin',(0.,-1.,0.));
#17514=CARTESIAN_POINT('Origin',(0.,-1.,0.));
#17515=CARTESIAN_POINT('Origin',(0.,-1.,0.));
#17516=CARTESIAN_POINT('Origin',(0.,-1.,0.));
#17517=CARTESIAN_POINT('Origin',(0.,-1.,0.));
#17518=CARTESIAN_POINT('Origin',(0.,-1.,0.));
#17519=CARTESIAN_POINT('Origin',(0.,-1.,0.));
#17520=CARTESIAN_POINT('',(1.26571495954046,-1.,0.524276302340173));
#17521=CARTESIAN_POINT('Origin',(0.,-1.,0.));
#17522=CARTESIAN_POINT('',(0.739103626009029,-1.,0.306146745892072));
#17523=CARTESIAN_POINT('',(0.632857479770231,-1.,0.262138151170086));
#17524=CARTESIAN_POINT('',(0.765552268585767,-1.,0.23222774180357));
#17525=CARTESIAN_POINT('',(0.745715786653214,-1.,0.287666994869947));
#17526=CARTESIAN_POINT('',(0.784628224322584,-1.,0.156072257612903));
#17527=CARTESIAN_POINT('',(0.770321257519971,-1.,0.213188870755903));
#17528=CARTESIAN_POINT('',(0.796147781337758,-1.,0.0784137122636485));
#17529=CARTESIAN_POINT('',(0.787508113576378,-1.,0.136657621275589));
#17530=CARTESIAN_POINT('',(0.8,-1.,0.));
#17531=CARTESIAN_POINT('',(0.797110836003318,-1.,0.0588102841977364));
#17532=CARTESIAN_POINT('',(0.796147781337758,-1.,-0.0784137122636485));
#17533=CARTESIAN_POINT('',(0.799036945334439,-1.,-0.0196034280659122));
#17534=CARTESIAN_POINT('',(0.784628224322584,-1.,-0.156072257612903));
#17535=CARTESIAN_POINT('',(0.793267892083964,-1.,-0.0978283486009621));
#17536=CARTESIAN_POINT('',(0.765552268585767,-1.,-0.23222774180357));
#17537=CARTESIAN_POINT('',(0.77985923538838,-1.,-0.17511112866057));
#17538=CARTESIAN_POINT('',(0.739103626009029,-1.,-0.306146745892072));
#17539=CARTESIAN_POINT('',(0.758940107941583,-1.,-0.250707492825696));
#17540=CARTESIAN_POINT('',(1.26571495954046,-1.,-0.524276302340173));
#17541=CARTESIAN_POINT('',(0.369551813004515,-1.,-0.153073372946036));
#17542=CARTESIAN_POINT('',(-0.17882088334147,-1.,-1.35827946008212));
#17543=CARTESIAN_POINT('Origin',(0.,-1.,0.));
#17544=CARTESIAN_POINT('',(-0.104420953776041,-1.,-0.793155889099048));
#17545=CARTESIAN_POINT('',(-0.0894104416707352,-1.,-0.67913973004106));
#17546=CARTESIAN_POINT('',(-0.181661010427498,-1.,-0.779101583421867));
#17547=CARTESIAN_POINT('',(-0.123730967938905,-1.,-0.789642312679753));
#17548=CARTESIAN_POINT('',(-0.257151572242529,-1.,-0.757544103596085));
#17549=CARTESIAN_POINT('',(-0.200533650881256,-1.,-0.773712213465422));
#17550=CARTESIAN_POINT('',(-0.330165623843516,-1.,-0.728691059936941));
#17551=CARTESIAN_POINT('',(-0.275405085142776,-1.,-0.750330842681299));
#17552=CARTESIAN_POINT('',(-0.4,-1.,-0.692820323027551));
#17553=CARTESIAN_POINT('',(-0.347624217882637,-1.,-0.719723375709593));
#17554=CARTESIAN_POINT('',(-0.465982157494242,-1.,-0.650277347673292));
#17555=CARTESIAN_POINT('',(-0.41649553937356,-1.,-0.682184579188986));
#17556=CARTESIAN_POINT('',(-0.527476652080055,-1.,-0.601471845983182));
#17557=CARTESIAN_POINT('',(-0.481355781140695,-1.,-0.638075972250765));
#17558=CARTESIAN_POINT('',(-0.583891258158268,-1.,-0.546873841618297));
#17559=CARTESIAN_POINT('',(-0.541580303599609,-1.,-0.587822344891961));
#17560=CARTESIAN_POINT('',(-0.634682672232988,-1.,-0.487009143206977));
#17561=CARTESIAN_POINT('',(-0.596589111676948,-1.,-0.531907667015467));
#17562=CARTESIAN_POINT('',(-1.08689407619899,-1.,-0.834003157741947));
#17563=CARTESIAN_POINT('',(-0.317341336116494,-1.,-0.243504571603488));
#17564=CARTESIAN_POINT('',(-1.37,-1.,-1.67776611483187E-16));
#17565=CARTESIAN_POINT('Origin',(0.,-1.,0.));
#17566=CARTESIAN_POINT('Origin',(0.,-1.,0.));
#17567=CARTESIAN_POINT('Origin',(-0.311094480357091,-0.4,-1.33421146160995));
#17568=CARTESIAN_POINT('',(-0.17882088334147,-0.4,-1.35827946008212));
#17569=CARTESIAN_POINT('',(-0.311094480357091,-0.4,-1.33421146160995));
#17570=CARTESIAN_POINT('',(-0.17882088334147,-0.4,-1.35827946008212));
#17571=CARTESIAN_POINT('',(-0.17882088334147,-0.4,-1.35827946008212));
#17572=CARTESIAN_POINT('',(-0.311094480357091,-1.,-1.33421146160995));
#17573=CARTESIAN_POINT('',(-0.278026081103185,-1.,-1.34022846122799));
#17574=CARTESIAN_POINT('',(-0.311094480357091,-0.4,-1.33421146160995));
#17575=CARTESIAN_POINT('Origin',(-0.440372067465331,-0.4,-1.29729427740829));
#17576=CARTESIAN_POINT('',(-0.440372067465331,-0.4,-1.29729427740829));
#17577=CARTESIAN_POINT('',(-0.311094480357091,-0.4,-1.33421146160995));
#17578=CARTESIAN_POINT('',(-0.440372067465331,-1.,-1.29729427740829));
#17579=CARTESIAN_POINT('',(-0.408052670688271,-1.,-1.30652357345871));
#17580=CARTESIAN_POINT('',(-0.440372067465331,-0.4,-1.29729427740829));
#17581=CARTESIAN_POINT('Origin',(-0.565408630832021,-0.4,-1.24788344014201));
#17582=CARTESIAN_POINT('',(-0.565408630832021,-0.4,-1.24788344014201));
#17583=CARTESIAN_POINT('',(-0.440372067465331,-0.4,-1.29729427740829));
#17584=CARTESIAN_POINT('',(-0.565408630832021,-1.,-1.24788344014201));
#17585=CARTESIAN_POINT('',(-0.534149489990348,-1.,-1.26023614945858));
#17586=CARTESIAN_POINT('',(-0.565408630832021,-0.4,-1.24788344014201));
#17587=CARTESIAN_POINT('Origin',(-0.685,-0.4,-1.18645480318468));
#17588=CARTESIAN_POINT('',(-0.685,-0.4,-1.18645480318468));
#17589=CARTESIAN_POINT('',(-0.565408630832021,-0.4,-1.24788344014201));
#17590=CARTESIAN_POINT('',(-0.685,-1.,-1.18645480318468));
#17591=CARTESIAN_POINT('',(-0.655102157708006,-1.,-1.20181196242401));
#17592=CARTESIAN_POINT('',(-0.685,-0.4,-1.18645480318468));
#17593=CARTESIAN_POINT('Origin',(-0.797994444708889,-0.4,-1.11359995789051));
#17594=CARTESIAN_POINT('',(-0.797994444708889,-0.4,-1.11359995789051));
#17595=CARTESIAN_POINT('',(-0.685,-0.4,-1.18645480318468));
#17596=CARTESIAN_POINT('',(-0.797994444708889,-1.,-1.11359995789051));
#17597=CARTESIAN_POINT('',(-0.769745833531665,-1.,-1.13181366921406));
#17598=CARTESIAN_POINT('',(-0.797994444708889,-0.4,-1.11359995789051));
#17599=CARTESIAN_POINT('Origin',(-0.903303766687094,-0.4,-1.0300205362462));
#17600=CARTESIAN_POINT('',(-0.903303766687094,-0.4,-1.0300205362462));
#17601=CARTESIAN_POINT('',(-0.797994444708889,-0.4,-1.11359995789051));
#17602=CARTESIAN_POINT('',(-0.903303766687094,-1.,-1.0300205362462));
#17603=CARTESIAN_POINT('',(-0.876976436192543,-1.,-1.05091539165728));
#17604=CARTESIAN_POINT('',(-0.903303766687094,-0.4,-1.0300205362462));
#17605=CARTESIAN_POINT('Origin',(-0.999913779596035,-0.4,-0.936521453771334));
#17606=CARTESIAN_POINT('',(-0.999913779596035,-0.4,-0.936521453771334));
#17607=CARTESIAN_POINT('',(-0.903303766687094,-0.4,-1.0300205362462));
#17608=CARTESIAN_POINT('',(-0.999913779596034,-1.,-0.936521453771334));
#17609=CARTESIAN_POINT('',(-0.9757612763688,-1.,-0.95989622439005));
#17610=CARTESIAN_POINT('',(-0.999913779596035,-0.4,-0.936521453771334));
#17611=CARTESIAN_POINT('Origin',(-1.08689407619899,-0.4,-0.834003157741947));
#17612=CARTESIAN_POINT('',(-1.08689407619899,-0.4,-0.834003157741947));
#17613=CARTESIAN_POINT('',(-0.999913779596035,-0.4,-0.936521453771334));
#17614=CARTESIAN_POINT('',(-1.06514900204825,-1.,-0.859632731749293));
#17615=CARTESIAN_POINT('',(-1.08689407619899,-0.4,-0.834003157741947));
#17616=CARTESIAN_POINT('Origin',(-0.634682672232988,-0.4,-0.487009143206977));
#17617=CARTESIAN_POINT('',(-0.634682672232988,-0.4,-0.487009143206977));
#17618=CARTESIAN_POINT('',(-1.08689407619899,-0.4,-0.834003157741947));
#17619=CARTESIAN_POINT('',(-0.634682672232988,-0.4,-0.487009143206977));
#17620=CARTESIAN_POINT('Origin',(-0.583891258158268,-0.4,-0.546873841618297));
#17621=CARTESIAN_POINT('',(-0.583891258158268,-0.4,-0.546873841618297));
#17622=CARTESIAN_POINT('',(-0.634682672232988,-0.4,-0.487009143206977));
#17623=CARTESIAN_POINT('',(-0.583891258158268,-0.4,-0.546873841618297));
#17624=CARTESIAN_POINT('Origin',(-0.527476652080055,-0.4,-0.601471845983182));
#17625=CARTESIAN_POINT('',(-0.527476652080055,-0.4,-0.601471845983182));
#17626=CARTESIAN_POINT('',(-0.583891258158268,-0.4,-0.546873841618297));
#17627=CARTESIAN_POINT('',(-0.527476652080055,-0.4,-0.601471845983182));
#17628=CARTESIAN_POINT('Origin',(-0.465982157494242,-0.4,-0.650277347673292));
#17629=CARTESIAN_POINT('',(-0.465982157494242,-0.4,-0.650277347673292));
#17630=CARTESIAN_POINT('',(-0.527476652080055,-0.4,-0.601471845983182));
#17631=CARTESIAN_POINT('',(-0.465982157494242,-0.4,-0.650277347673292));
#17632=CARTESIAN_POINT('Origin',(-0.4,-0.4,-0.692820323027551));
#17633=CARTESIAN_POINT('',(-0.4,-0.4,-0.692820323027551));
#17634=CARTESIAN_POINT('',(-0.465982157494242,-0.4,-0.650277347673292));
#17635=CARTESIAN_POINT('',(-0.4,-0.4,-0.692820323027551));
#17636=CARTESIAN_POINT('Origin',(-0.330165623843516,-0.4,-0.728691059936941));
#17637=CARTESIAN_POINT('',(-0.330165623843516,-0.4,-0.728691059936941));
#17638=CARTESIAN_POINT('',(-0.4,-0.4,-0.692820323027551));
#17639=CARTESIAN_POINT('',(-0.330165623843516,-0.4,-0.728691059936941));
#17640=CARTESIAN_POINT('Origin',(-0.257151572242529,-0.4,-0.757544103596085));
#17641=CARTESIAN_POINT('',(-0.257151572242529,-0.4,-0.757544103596085));
#17642=CARTESIAN_POINT('',(-0.330165623843516,-0.4,-0.728691059936941));
#17643=CARTESIAN_POINT('',(-0.257151572242529,-0.4,-0.757544103596085));
#17644=CARTESIAN_POINT('Origin',(-0.181661010427498,-0.4,-0.779101583421867));
#17645=CARTESIAN_POINT('',(-0.181661010427498,-0.4,-0.779101583421867));
#17646=CARTESIAN_POINT('',(-0.257151572242529,-0.4,-0.757544103596085));
#17647=CARTESIAN_POINT('',(-0.181661010427498,-0.4,-0.779101583421867));
#17648=CARTESIAN_POINT('Origin',(-0.104420953776041,-0.4,-0.793155889099048));
#17649=CARTESIAN_POINT('',(-0.104420953776041,-0.4,-0.793155889099048));
#17650=CARTESIAN_POINT('',(-0.181661010427498,-0.4,-0.779101583421867));
#17651=CARTESIAN_POINT('',(-0.104420953776041,-0.4,-0.793155889099048));
#17652=CARTESIAN_POINT('Origin',(-0.17882088334147,-0.4,-1.35827946008212));
#17653=CARTESIAN_POINT('',(-0.104420953776041,-0.4,-0.793155889099048));
#17654=CARTESIAN_POINT('Origin',(-0.527275906502257,-0.4,-0.913268659668847));
#17655=CARTESIAN_POINT('Origin',(0.,-1.,0.));
#17656=CARTESIAN_POINT('Origin',(0.,-1.,0.));
#17657=CARTESIAN_POINT('Origin',(0.,-1.,0.));
#17658=CARTESIAN_POINT('Origin',(0.,-1.,0.));
#17659=CARTESIAN_POINT('Origin',(0.,-1.,0.));
#17660=CARTESIAN_POINT('Origin',(0.,-1.,0.));
#17661=CARTESIAN_POINT('Origin',(0.,-1.,0.));
#17662=CARTESIAN_POINT('Origin',(0.,-1.,0.));
#17663=CARTESIAN_POINT('Origin',(0.,-1.,0.));
#17664=CARTESIAN_POINT('Origin',(0.,-1.,0.));
#17665=CARTESIAN_POINT('Origin',(0.,-1.,0.));
#17666=CARTESIAN_POINT('Origin',(0.,-1.,0.));
#17667=CARTESIAN_POINT('Origin',(0.,-1.,0.));
#17668=CARTESIAN_POINT('Origin',(0.,-1.,0.));
#17669=CARTESIAN_POINT('Origin',(0.,-1.,0.));
#17670=CARTESIAN_POINT('Origin',(0.,-1.,0.));
#17671=CARTESIAN_POINT('Origin',(1.31100825995313,-0.4,0.397690007838613));
#17672=CARTESIAN_POINT('',(1.26571495954046,-0.4,0.524276302340173));
#17673=CARTESIAN_POINT('',(1.31100825995313,-0.4,0.397690007838613));
#17674=CARTESIAN_POINT('',(1.26571495954046,-0.4,0.524276302340173));
#17675=CARTESIAN_POINT('',(1.26571495954046,-0.4,0.524276302340173));
#17676=CARTESIAN_POINT('',(1.31100825995313,-1.,0.397690007838613));
#17677=CARTESIAN_POINT('',(1.29968493484996,-1.,0.429336581464004));
#17678=CARTESIAN_POINT('',(1.31100825995313,-0.4,0.397690007838613));
#17679=CARTESIAN_POINT('Origin',(1.34367583415243,-0.4,0.267273741162096));
#17680=CARTESIAN_POINT('',(1.34367583415243,-0.4,0.267273741162096));
#17681=CARTESIAN_POINT('',(1.31100825995313,-0.4,0.397690007838613));
#17682=CARTESIAN_POINT('',(1.34367583415243,-1.,0.267273741162096));
#17683=CARTESIAN_POINT('',(1.3355089406026,-1.,0.299877807831226));
#17684=CARTESIAN_POINT('',(1.34367583415243,-0.4,0.267273741162096));
#17685=CARTESIAN_POINT('Origin',(1.36340307554091,-0.4,0.134283482251498));
#17686=CARTESIAN_POINT('',(1.36340307554091,-0.4,0.134283482251498));
#17687=CARTESIAN_POINT('',(1.34367583415243,-0.4,0.267273741162096));
#17688=CARTESIAN_POINT('',(1.36340307554091,-1.,0.134283482251498));
#17689=CARTESIAN_POINT('',(1.35847126519379,-1.,0.167531046979148));
#17690=CARTESIAN_POINT('',(1.36340307554091,-0.4,0.134283482251498));
#17691=CARTESIAN_POINT('Origin',(1.37,-0.4,0.));
#17692=CARTESIAN_POINT('',(1.37,-0.4,0.));
#17693=CARTESIAN_POINT('',(1.36340307554091,-0.4,0.134283482251498));
#17694=CARTESIAN_POINT('',(1.37,-1.,0.));
#17695=CARTESIAN_POINT('',(1.36835076888523,-1.,0.0335708705628731));
#17696=CARTESIAN_POINT('',(1.37,-0.4,0.));
#17697=CARTESIAN_POINT('Origin',(1.36340307554091,-0.4,-0.134283482251498));
#17698=CARTESIAN_POINT('',(1.36340307554091,-0.4,-0.134283482251498));
#17699=CARTESIAN_POINT('',(1.37,-0.4,0.));
#17700=CARTESIAN_POINT('',(1.36340307554091,-1.,-0.134283482251498));
#17701=CARTESIAN_POINT('',(1.36505230665568,-1.,-0.100712611688622));
#17702=CARTESIAN_POINT('',(1.36340307554091,-0.4,-0.134283482251498));
#17703=CARTESIAN_POINT('Origin',(1.34367583415243,-0.4,-0.267273741162096));
#17704=CARTESIAN_POINT('',(1.34367583415243,-0.4,-0.267273741162096));
#17705=CARTESIAN_POINT('',(1.36340307554091,-0.4,-0.134283482251498));
#17706=CARTESIAN_POINT('',(1.34367583415243,-1.,-0.267273741162096));
#17707=CARTESIAN_POINT('',(1.34860764449955,-1.,-0.234026176434447));
#17708=CARTESIAN_POINT('',(1.34367583415243,-0.4,-0.267273741162096));
#17709=CARTESIAN_POINT('Origin',(1.31100825995313,-0.4,-0.397690007838613));
#17710=CARTESIAN_POINT('',(1.31100825995313,-0.4,-0.397690007838613));
#17711=CARTESIAN_POINT('',(1.34367583415243,-0.4,-0.267273741162096));
#17712=CARTESIAN_POINT('',(1.31100825995313,-1.,-0.397690007838613));
#17713=CARTESIAN_POINT('',(1.31917515350295,-1.,-0.365085941169485));
#17714=CARTESIAN_POINT('',(1.31100825995313,-0.4,-0.397690007838613));
#17715=CARTESIAN_POINT('Origin',(1.26571495954046,-0.4,-0.524276302340173));
#17716=CARTESIAN_POINT('',(1.26571495954046,-0.4,-0.524276302340173));
#17717=CARTESIAN_POINT('',(1.31100825995313,-0.4,-0.397690007838613));
#17718=CARTESIAN_POINT('',(1.27703828464363,-1.,-0.492629728714784));
#17719=CARTESIAN_POINT('',(1.26571495954046,-0.4,-0.524276302340173));
#17720=CARTESIAN_POINT('Origin',(0.739103626009029,-0.4,-0.306146745892072));
#17721=CARTESIAN_POINT('',(0.739103626009029,-0.4,-0.306146745892072));
#17722=CARTESIAN_POINT('',(1.26571495954046,-0.4,-0.524276302340173));
#17723=CARTESIAN_POINT('',(0.739103626009029,-0.4,-0.306146745892072));
#17724=CARTESIAN_POINT('Origin',(0.765552268585767,-0.4,-0.23222774180357));
#17725=CARTESIAN_POINT('',(0.765552268585767,-0.4,-0.23222774180357));
#17726=CARTESIAN_POINT('',(0.739103626009029,-0.4,-0.306146745892072));
#17727=CARTESIAN_POINT('',(0.765552268585767,-0.4,-0.23222774180357));
#17728=CARTESIAN_POINT('Origin',(0.784628224322584,-0.4,-0.156072257612903));
#17729=CARTESIAN_POINT('',(0.784628224322584,-0.4,-0.156072257612903));
#17730=CARTESIAN_POINT('',(0.765552268585767,-0.4,-0.23222774180357));
#17731=CARTESIAN_POINT('',(0.784628224322584,-0.4,-0.156072257612903));
#17732=CARTESIAN_POINT('Origin',(0.796147781337758,-0.4,-0.0784137122636485));
#17733=CARTESIAN_POINT('',(0.796147781337758,-0.4,-0.0784137122636485));
#17734=CARTESIAN_POINT('',(0.784628224322584,-0.4,-0.156072257612903));
#17735=CARTESIAN_POINT('',(0.796147781337758,-0.4,-0.0784137122636485));
#17736=CARTESIAN_POINT('Origin',(0.8,-0.4,0.));
#17737=CARTESIAN_POINT('',(0.8,-0.4,0.));
#17738=CARTESIAN_POINT('',(0.796147781337758,-0.4,-0.0784137122636485));
#17739=CARTESIAN_POINT('',(0.8,-0.4,0.));
#17740=CARTESIAN_POINT('Origin',(0.796147781337758,-0.4,0.0784137122636485));
#17741=CARTESIAN_POINT('',(0.796147781337758,-0.4,0.0784137122636485));
#17742=CARTESIAN_POINT('',(0.8,-0.4,0.));
#17743=CARTESIAN_POINT('',(0.796147781337758,-0.4,0.0784137122636485));
#17744=CARTESIAN_POINT('Origin',(0.784628224322584,-0.4,0.156072257612903));
#17745=CARTESIAN_POINT('',(0.784628224322584,-0.4,0.156072257612903));
#17746=CARTESIAN_POINT('',(0.796147781337758,-0.4,0.0784137122636485));
#17747=CARTESIAN_POINT('',(0.784628224322584,-0.4,0.156072257612903));
#17748=CARTESIAN_POINT('Origin',(0.765552268585767,-0.4,0.23222774180357));
#17749=CARTESIAN_POINT('',(0.765552268585767,-0.4,0.23222774180357));
#17750=CARTESIAN_POINT('',(0.784628224322584,-0.4,0.156072257612903));
#17751=CARTESIAN_POINT('',(0.765552268585767,-0.4,0.23222774180357));
#17752=CARTESIAN_POINT('Origin',(0.739103626009029,-0.4,0.306146745892072));
#17753=CARTESIAN_POINT('',(0.739103626009029,-0.4,0.306146745892072));
#17754=CARTESIAN_POINT('',(0.765552268585767,-0.4,0.23222774180357));
#17755=CARTESIAN_POINT('',(0.739103626009029,-0.4,0.306146745892072));
#17756=CARTESIAN_POINT('Origin',(1.26571495954046,-0.4,0.524276302340173));
#17757=CARTESIAN_POINT('',(0.739103626009029,-0.4,0.306146745892072));
#17758=CARTESIAN_POINT('Origin',(1.05455181300451,-0.4,0.));
#17759=CARTESIAN_POINT('Origin',(0.,-1.,0.));
#17760=CARTESIAN_POINT('Origin',(0.,-1.,0.));
#17761=CARTESIAN_POINT('Origin',(0.,-1.,0.));
#17762=CARTESIAN_POINT('Origin',(0.,-1.,0.));
#17763=CARTESIAN_POINT('Origin',(0.,-1.,0.));
#17764=CARTESIAN_POINT('Origin',(0.,-1.,0.));
#17765=CARTESIAN_POINT('Origin',(0.,-1.,0.));
#17766=CARTESIAN_POINT('Origin',(0.,-1.,0.));
#17767=CARTESIAN_POINT('Origin',(0.,-1.,0.));
#17768=CARTESIAN_POINT('Origin',(0.,-1.,0.));
#17769=CARTESIAN_POINT('Origin',(0.,-1.,0.));
#17770=CARTESIAN_POINT('Origin',(0.,-1.,0.));
#17771=CARTESIAN_POINT('Origin',(0.,-1.,0.));
#17772=CARTESIAN_POINT('Origin',(0.,-1.,0.));
#17773=CARTESIAN_POINT('Origin',(0.,-1.,0.));
#17774=CARTESIAN_POINT('Origin',(0.,-1.,0.));
#17775=CARTESIAN_POINT('Origin',(0.,-1.,0.));
#17776=CARTESIAN_POINT('',(-1.37,-2.05,1.67776611483187E-16));
#17777=CARTESIAN_POINT('Origin',(0.,-2.05,0.));
#17778=CARTESIAN_POINT('',(-1.37,-1.,-1.67776611483187E-16));
#17779=CARTESIAN_POINT('Origin',(0.,-2.05,0.));
#19317=UNCERTAINTY_MEASURE_WITH_UNIT(LENGTH_MEASURE(0.001),#19362,
'DISTANCE_ACCURACY_VALUE',
'Maximum model space distance between geometric entities at asserted c
onnectivities');
#19323=UNCERTAINTY_MEASURE_WITH_UNIT(LENGTH_MEASURE(0.001),#19362,
'DISTANCE_ACCURACY_VALUE',
'Maximum model space distance between geometric entities at asserted c
onnectivities');
#19355=(
GEOMETRIC_REPRESENTATION_CONTEXT(3)
GLOBAL_UNCERTAINTY_ASSIGNED_CONTEXT((#19317))
GLOBAL_UNIT_ASSIGNED_CONTEXT((#19362,#19364,#19365))
REPRESENTATION_CONTEXT('','3D')
);
#19361=(
GEOMETRIC_REPRESENTATION_CONTEXT(3)
GLOBAL_UNCERTAINTY_ASSIGNED_CONTEXT((#19323))
GLOBAL_UNIT_ASSIGNED_CONTEXT((#19362,#19364,#19365))
REPRESENTATION_CONTEXT('','3D')
);
#19362=(
LENGTH_UNIT()
NAMED_UNIT(*)
SI_UNIT(.CENTI.,.METRE.)
);
#19364=(
NAMED_UNIT(*)
PLANE_ANGLE_UNIT()
SI_UNIT($,.RADIAN.)
);
#19365=(
NAMED_UNIT(*)
SI_UNIT($,.STERADIAN.)
SOLID_ANGLE_UNIT()
);
#19397=SHAPE_DEFINITION_REPRESENTATION(#19461,#19519);
#19461=PRODUCT_DEFINITION_SHAPE('',$,#19557);
#19519=SHAPE_REPRESENTATION('',(#11864),#19355);
#19525=PRODUCT_DEFINITION_CONTEXT('part definition',#19638,'design');
#19557=PRODUCT_DEFINITION('Hub A','Hub A',#19594,#19525);
#19594=PRODUCT_DEFINITION_FORMATION('',$,#19671);
#19638=APPLICATION_CONTEXT(
'Core Data for Automotive Mechanical Design Process');
#19639=PRODUCT_CONTEXT('part definition',#19638,'mechanical');
#19671=PRODUCT('Hub A','Hub A','Hub A',(#19639));
#19733=COLOUR_RGB('Sky Blue',0.24,0.69,0.87);
#19734=FILL_AREA_STYLE_COLOUR('',#19733);
#19735=FILL_AREA_STYLE('',(#19734));
#19736=SURFACE_STYLE_FILL_AREA(#19735);
#19737=SURFACE_SIDE_STYLE('',(#19736));
#19738=SURFACE_STYLE_USAGE(.BOTH.,#19737);
#19739=PRESENTATION_STYLE_ASSIGNMENT((#19738));
ENDSEC;
END-ISO-10303-21;
